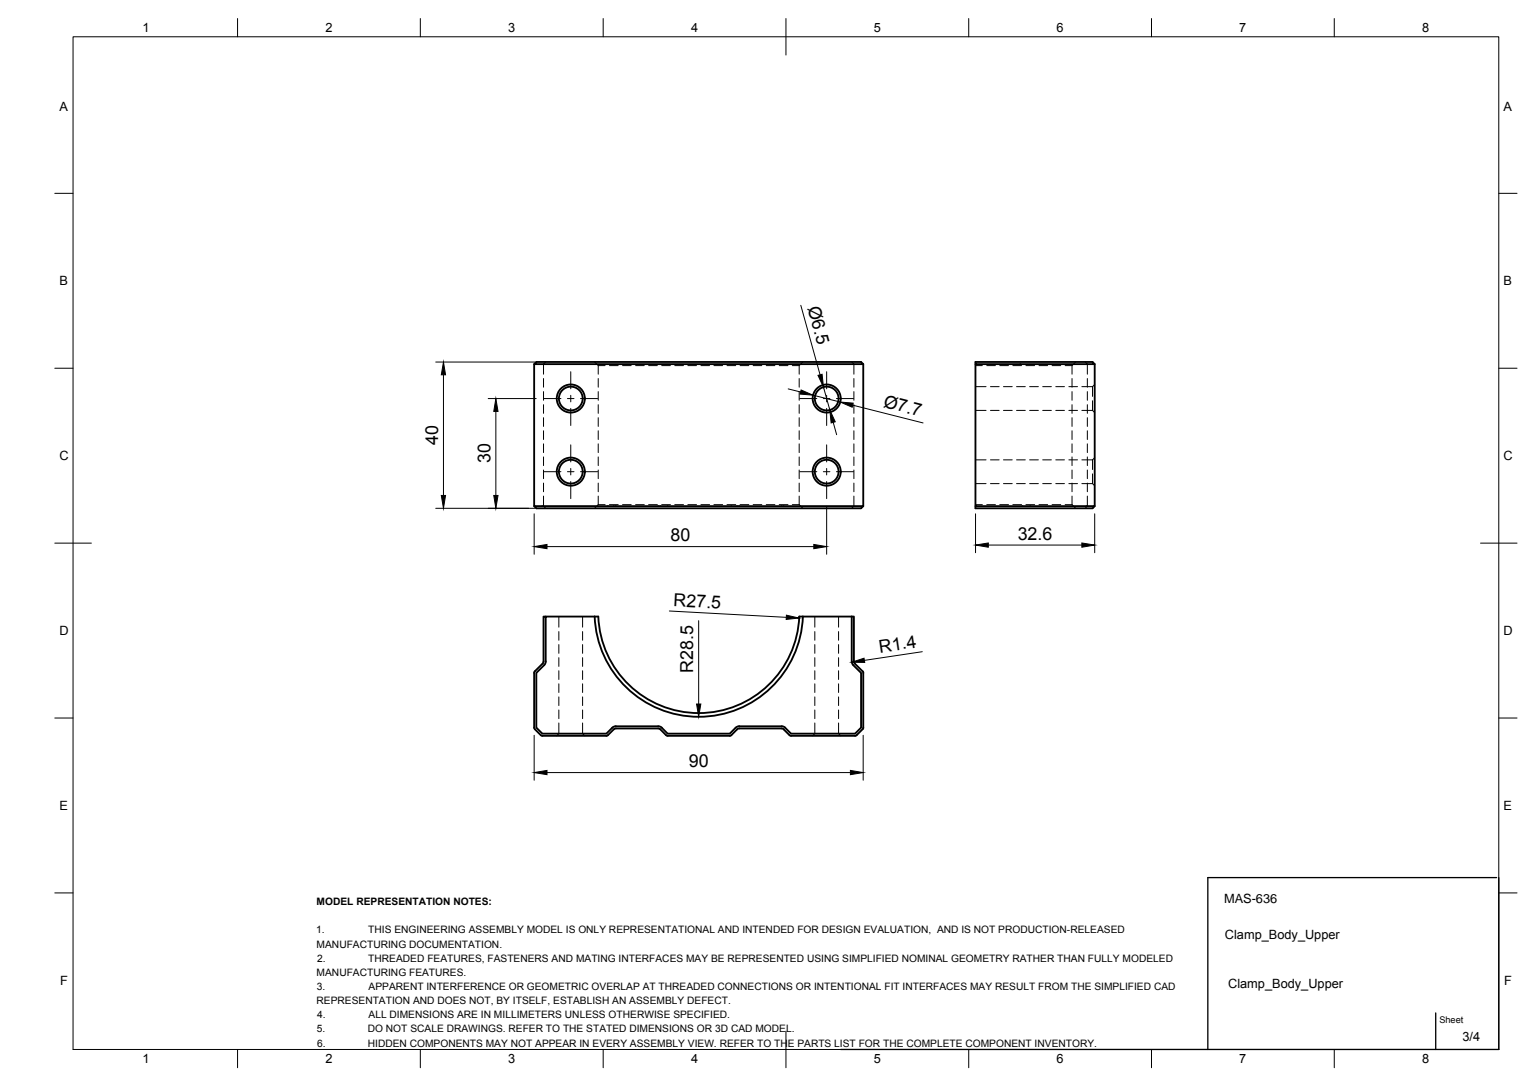
ISO-10303-21;
HEADER;
FILE_DESCRIPTION((''),'2;1');
FILE_NAME('Clamp_Body_Upper.step','2026-10-09T10:15:02-07:00',(''),(''),'','','');
FILE_SCHEMA (('AUTOMOTIVE_DESIGN { 1 0 10303 214 3 1 1 }'));
ENDSEC;
DATA;
#10=MECHANICAL_DESIGN_GEOMETRIC_PRESENTATION_REPRESENTATION('',(#83),#6779);
#63=SHAPE_REPRESENTATION_RELATIONSHIP('SRR','None',#6817,#73) ;
#73=ADVANCED_BREP_SHAPE_REPRESENTATION('',(#93),#6769) ;
#83=STYLED_ITEM('',(#6876),#93) ;
#93=MANIFOLD_SOLID_BREP('Body1',#3895) ;
#103=FACE_BOUND('',#628,.T.) ;
#104=FACE_BOUND('',#629,.T.) ;
#105=FACE_BOUND('',#631,.T.) ;
#106=FACE_BOUND('',#632,.T.) ;
#107=FACE_BOUND('',#638,.T.) ;
#108=FACE_BOUND('',#639,.T.) ;
#109=FACE_BOUND('',#649,.T.) ;
#110=FACE_BOUND('',#650,.T.) ;
#135=PLANE('',#4045) ;
#136=PLANE('',#4054) ;
#137=PLANE('',#4057) ;
#138=PLANE('',#4060) ;
#139=PLANE('',#4063) ;
#140=PLANE('',#4066) ;
#141=PLANE('',#4069) ;
#142=PLANE('',#4072) ;
#143=PLANE('',#4075) ;
#144=PLANE('',#4078) ;
#145=PLANE('',#4081) ;
#146=PLANE('',#4084) ;
#147=PLANE('',#4087) ;
#148=PLANE('',#4090) ;
#149=PLANE('',#4093) ;
#150=PLANE('',#4096) ;
#151=PLANE('',#4099) ;
#152=PLANE('',#4100) ;
#153=PLANE('',#4101) ;
#154=PLANE('',#4120) ;
#155=PLANE('',#4121) ;
#156=PLANE('',#4122) ;
#157=PLANE('',#4123) ;
#158=PLANE('',#4124) ;
#159=PLANE('',#4125) ;
#160=PLANE('',#4128) ;
#161=PLANE('',#4131) ;
#162=PLANE('',#4132) ;
#163=PLANE('',#4135) ;
#164=PLANE('',#4138) ;
#165=PLANE('',#4139) ;
#166=PLANE('',#4142) ;
#167=PLANE('',#4145) ;
#168=PLANE('',#4148) ;
#169=PLANE('',#4151) ;
#170=PLANE('',#4152) ;
#171=PLANE('',#4155) ;
#172=PLANE('',#4156) ;
#173=PLANE('',#4160) ;
#174=PLANE('',#4162) ;
#175=PLANE('',#4164) ;
#176=PLANE('',#4166) ;
#177=PLANE('',#4168) ;
#178=PLANE('',#4170) ;
#179=PLANE('',#4172) ;
#180=PLANE('',#4174) ;
#181=PLANE('',#4176) ;
#182=PLANE('',#4178) ;
#183=PLANE('',#4180) ;
#184=PLANE('',#4182) ;
#185=PLANE('',#4184) ;
#186=PLANE('',#4186) ;
#187=PLANE('',#4188) ;
#188=PLANE('',#4190) ;
#189=PLANE('',#4191) ;
#263=(
BOUNDED_CURVE()
B_SPLINE_CURVE(2,(#5652,#5653,#5654),.UNSPECIFIED.,.F.,.F.)
B_SPLINE_CURVE_WITH_KNOTS((3,3),(8.17571637705571,8.18145882895963),
 .UNSPECIFIED.)
CURVE()
GEOMETRIC_REPRESENTATION_ITEM()
RATIONAL_B_SPLINE_CURVE((1.06993006993377,1.0518696293833,1.03378378378363))
REPRESENTATION_ITEM('')
) ;
#264=(
BOUNDED_CURVE()
B_SPLINE_CURVE(2,(#5656,#5657,#5658),.UNSPECIFIED.,.F.,.F.)
B_SPLINE_CURVE_WITH_KNOTS((3,3),(-0.0111022969227764,-0.00535984501964869),
 .UNSPECIFIED.)
CURVE()
GEOMETRIC_REPRESENTATION_ITEM()
RATIONAL_B_SPLINE_CURVE((1.06993006993377,1.0518696293858,1.03378378378863))
REPRESENTATION_ITEM('')
) ;
#265=(
BOUNDED_CURVE()
B_SPLINE_CURVE(2,(#5664,#5665,#5666),.UNSPECIFIED.,.F.,.F.)
B_SPLINE_CURVE_WITH_KNOTS((3,3),(8.1757163770557,8.18145882895962),
 .UNSPECIFIED.)
CURVE()
GEOMETRIC_REPRESENTATION_ITEM()
RATIONAL_B_SPLINE_CURVE((1.06993006993376,1.05186962938329,1.03378378378362))
REPRESENTATION_ITEM('')
) ;
#266=(
BOUNDED_CURVE()
B_SPLINE_CURVE(2,(#5667,#5668,#5669),.UNSPECIFIED.,.F.,.F.)
B_SPLINE_CURVE_WITH_KNOTS((3,3),(-0.0111022969227769,-0.00535984501964911),
 .UNSPECIFIED.)
CURVE()
GEOMETRIC_REPRESENTATION_ITEM()
RATIONAL_B_SPLINE_CURVE((1.06993006993377,1.0518696293858,1.03378378378863))
REPRESENTATION_ITEM('')
) ;
#267=CONICAL_SURFACE('',#4021,1.,0.785398163397) ;
#268=CONICAL_SURFACE('',#4023,1.,0.785398163397) ;
#269=CONICAL_SURFACE('',#4028,1.,0.785398163398) ;
#270=CONICAL_SURFACE('',#4033,1.,0.785398163398) ;
#271=CONICAL_SURFACE('',#4038,1.,0.785398163398) ;
#272=CONICAL_SURFACE('',#4043,1.,0.785398163398) ;
#273=CONICAL_SURFACE('',#4052,1.,0.785398163392) ;
#274=CONICAL_SURFACE('',#4055,1.,0.785398163397) ;
#275=CONICAL_SURFACE('',#4058,1.,0.785398163397) ;
#276=CONICAL_SURFACE('',#4061,1.,0.785398163397) ;
#277=CONICAL_SURFACE('',#4064,1.,0.785398163397) ;
#278=CONICAL_SURFACE('',#4067,1.,0.785398163392) ;
#279=CONICAL_SURFACE('',#4070,1.,0.785398163392) ;
#280=CONICAL_SURFACE('',#4073,1.,0.785398163397) ;
#281=CONICAL_SURFACE('',#4076,1.,0.785398163397) ;
#282=CONICAL_SURFACE('',#4079,1.,0.785398163397) ;
#283=CONICAL_SURFACE('',#4082,1.,0.785398163397) ;
#284=CONICAL_SURFACE('',#4085,1.,0.785398163397) ;
#285=CONICAL_SURFACE('',#4088,1.,0.785398163397) ;
#286=CONICAL_SURFACE('',#4091,1.,0.785398163397) ;
#287=CONICAL_SURFACE('',#4094,1.,0.785398163397) ;
#288=CONICAL_SURFACE('',#4097,1.,0.785398163397) ;
#289=CONICAL_SURFACE('',#4159,1.,0.785398163392) ;
#290=CONICAL_SURFACE('',#4161,1.,0.785398163397) ;
#291=CONICAL_SURFACE('',#4163,1.,0.785398163397) ;
#292=CONICAL_SURFACE('',#4165,1.,0.785398163397) ;
#293=CONICAL_SURFACE('',#4167,1.,0.785398163397) ;
#294=CONICAL_SURFACE('',#4169,1.,0.785398163372) ;
#295=CONICAL_SURFACE('',#4171,1.,0.785398163372) ;
#296=CONICAL_SURFACE('',#4173,1.,0.785398163397) ;
#297=CONICAL_SURFACE('',#4175,1.,0.785398163397) ;
#298=CONICAL_SURFACE('',#4177,1.,0.785398163397) ;
#299=CONICAL_SURFACE('',#4179,1.,0.785398163397) ;
#300=CONICAL_SURFACE('',#4181,1.,0.785398163397) ;
#301=CONICAL_SURFACE('',#4183,1.,0.785398163397) ;
#302=CONICAL_SURFACE('',#4185,1.,0.785398163397) ;
#303=CONICAL_SURFACE('',#4187,1.,0.785398163397) ;
#304=CONICAL_SURFACE('',#4189,1.,0.785398163397) ;
#327=FACE_OUTER_BOUND('',#571,.T.) ;
#328=FACE_OUTER_BOUND('',#572,.T.) ;
#329=FACE_OUTER_BOUND('',#573,.T.) ;
#330=FACE_OUTER_BOUND('',#574,.T.) ;
#331=FACE_OUTER_BOUND('',#575,.T.) ;
#332=FACE_OUTER_BOUND('',#576,.T.) ;
#333=FACE_OUTER_BOUND('',#577,.T.) ;
#334=FACE_OUTER_BOUND('',#578,.T.) ;
#335=FACE_OUTER_BOUND('',#579,.T.) ;
#336=FACE_OUTER_BOUND('',#580,.T.) ;
#337=FACE_OUTER_BOUND('',#581,.T.) ;
#338=FACE_OUTER_BOUND('',#582,.T.) ;
#339=FACE_OUTER_BOUND('',#583,.T.) ;
#340=FACE_OUTER_BOUND('',#584,.T.) ;
#341=FACE_OUTER_BOUND('',#585,.T.) ;
#342=FACE_OUTER_BOUND('',#586,.T.) ;
#343=FACE_OUTER_BOUND('',#587,.T.) ;
#344=FACE_OUTER_BOUND('',#588,.T.) ;
#345=FACE_OUTER_BOUND('',#589,.T.) ;
#346=FACE_OUTER_BOUND('',#590,.T.) ;
#347=FACE_OUTER_BOUND('',#591,.T.) ;
#348=FACE_OUTER_BOUND('',#592,.T.) ;
#349=FACE_OUTER_BOUND('',#593,.T.) ;
#350=FACE_OUTER_BOUND('',#594,.T.) ;
#351=FACE_OUTER_BOUND('',#595,.T.) ;
#352=FACE_OUTER_BOUND('',#596,.T.) ;
#353=FACE_OUTER_BOUND('',#597,.T.) ;
#354=FACE_OUTER_BOUND('',#598,.T.) ;
#355=FACE_OUTER_BOUND('',#599,.T.) ;
#356=FACE_OUTER_BOUND('',#600,.T.) ;
#357=FACE_OUTER_BOUND('',#601,.T.) ;
#358=FACE_OUTER_BOUND('',#602,.T.) ;
#359=FACE_OUTER_BOUND('',#603,.T.) ;
#360=FACE_OUTER_BOUND('',#604,.T.) ;
#361=FACE_OUTER_BOUND('',#605,.T.) ;
#362=FACE_OUTER_BOUND('',#606,.T.) ;
#363=FACE_OUTER_BOUND('',#607,.T.) ;
#364=FACE_OUTER_BOUND('',#608,.T.) ;
#365=FACE_OUTER_BOUND('',#609,.T.) ;
#366=FACE_OUTER_BOUND('',#610,.T.) ;
#367=FACE_OUTER_BOUND('',#611,.T.) ;
#368=FACE_OUTER_BOUND('',#612,.T.) ;
#369=FACE_OUTER_BOUND('',#613,.T.) ;
#370=FACE_OUTER_BOUND('',#614,.T.) ;
#371=FACE_OUTER_BOUND('',#615,.T.) ;
#372=FACE_OUTER_BOUND('',#616,.T.) ;
#373=FACE_OUTER_BOUND('',#617,.T.) ;
#374=FACE_OUTER_BOUND('',#618,.T.) ;
#375=FACE_OUTER_BOUND('',#619,.T.) ;
#376=FACE_OUTER_BOUND('',#620,.T.) ;
#377=FACE_OUTER_BOUND('',#621,.T.) ;
#378=FACE_OUTER_BOUND('',#622,.T.) ;
#379=FACE_OUTER_BOUND('',#623,.T.) ;
#380=FACE_OUTER_BOUND('',#624,.T.) ;
#381=FACE_OUTER_BOUND('',#625,.T.) ;
#382=FACE_OUTER_BOUND('',#626,.T.) ;
#383=FACE_OUTER_BOUND('',#627,.T.) ;
#384=FACE_OUTER_BOUND('',#630,.T.) ;
#385=FACE_OUTER_BOUND('',#633,.T.) ;
#386=FACE_OUTER_BOUND('',#634,.T.) ;
#387=FACE_OUTER_BOUND('',#635,.T.) ;
#388=FACE_OUTER_BOUND('',#636,.T.) ;
#389=FACE_OUTER_BOUND('',#637,.T.) ;
#390=FACE_OUTER_BOUND('',#640,.T.) ;
#391=FACE_OUTER_BOUND('',#641,.T.) ;
#392=FACE_OUTER_BOUND('',#642,.T.) ;
#393=FACE_OUTER_BOUND('',#643,.T.) ;
#394=FACE_OUTER_BOUND('',#644,.T.) ;
#395=FACE_OUTER_BOUND('',#645,.T.) ;
#396=FACE_OUTER_BOUND('',#646,.T.) ;
#397=FACE_OUTER_BOUND('',#647,.T.) ;
#398=FACE_OUTER_BOUND('',#648,.T.) ;
#399=FACE_OUTER_BOUND('',#651,.T.) ;
#400=FACE_OUTER_BOUND('',#652,.T.) ;
#401=FACE_OUTER_BOUND('',#653,.T.) ;
#402=FACE_OUTER_BOUND('',#654,.T.) ;
#403=FACE_OUTER_BOUND('',#655,.T.) ;
#404=FACE_OUTER_BOUND('',#656,.T.) ;
#405=FACE_OUTER_BOUND('',#657,.T.) ;
#406=FACE_OUTER_BOUND('',#658,.T.) ;
#407=FACE_OUTER_BOUND('',#659,.T.) ;
#408=FACE_OUTER_BOUND('',#660,.T.) ;
#409=FACE_OUTER_BOUND('',#661,.T.) ;
#410=FACE_OUTER_BOUND('',#662,.T.) ;
#411=FACE_OUTER_BOUND('',#663,.T.) ;
#412=FACE_OUTER_BOUND('',#664,.T.) ;
#413=FACE_OUTER_BOUND('',#665,.T.) ;
#414=FACE_OUTER_BOUND('',#666,.T.) ;
#415=FACE_OUTER_BOUND('',#667,.T.) ;
#416=FACE_OUTER_BOUND('',#668,.T.) ;
#417=FACE_OUTER_BOUND('',#669,.T.) ;
#418=FACE_OUTER_BOUND('',#670,.T.) ;
#419=FACE_OUTER_BOUND('',#671,.T.) ;
#420=FACE_OUTER_BOUND('',#672,.T.) ;
#421=FACE_OUTER_BOUND('',#673,.T.) ;
#422=FACE_OUTER_BOUND('',#674,.T.) ;
#423=FACE_OUTER_BOUND('',#675,.T.) ;
#424=FACE_OUTER_BOUND('',#676,.T.) ;
#425=FACE_OUTER_BOUND('',#677,.T.) ;
#426=FACE_OUTER_BOUND('',#678,.T.) ;
#427=FACE_OUTER_BOUND('',#679,.T.) ;
#428=FACE_OUTER_BOUND('',#680,.T.) ;
#429=FACE_OUTER_BOUND('',#681,.T.) ;
#430=FACE_OUTER_BOUND('',#682,.T.) ;
#431=FACE_OUTER_BOUND('',#683,.T.) ;
#432=FACE_OUTER_BOUND('',#684,.T.) ;
#433=FACE_OUTER_BOUND('',#685,.T.) ;
#434=FACE_OUTER_BOUND('',#686,.T.) ;
#435=FACE_OUTER_BOUND('',#687,.T.) ;
#436=FACE_OUTER_BOUND('',#688,.T.) ;
#437=FACE_OUTER_BOUND('',#689,.T.) ;
#438=FACE_OUTER_BOUND('',#690,.T.) ;
#439=FACE_OUTER_BOUND('',#691,.T.) ;
#440=FACE_OUTER_BOUND('',#692,.T.) ;
#571=EDGE_LOOP('',(#2555,#2556,#2557,#2558)) ;
#572=EDGE_LOOP('',(#2559,#2560,#2561,#2562)) ;
#573=EDGE_LOOP('',(#2563,#2564,#2565,#2566)) ;
#574=EDGE_LOOP('',(#2567,#2568,#2569,#2570)) ;
#575=EDGE_LOOP('',(#2571,#2572,#2573,#2574)) ;
#576=EDGE_LOOP('',(#2575,#2576,#2577,#2578)) ;
#577=EDGE_LOOP('',(#2579,#2580,#2581,#2582)) ;
#578=EDGE_LOOP('',(#2583,#2584,#2585,#2586)) ;
#579=EDGE_LOOP('',(#2587,#2588,#2589,#2590)) ;
#580=EDGE_LOOP('',(#2591,#2592,#2593,#2594)) ;
#581=EDGE_LOOP('',(#2595,#2596,#2597,#2598)) ;
#582=EDGE_LOOP('',(#2599,#2600,#2601,#2602,#2603,#2604,#2605,#2606,#2607,
#2608,#2609,#2610,#2611,#2612,#2613,#2614,#2615,#2616,#2617,#2618,#2619,
#2620,#2621,#2622,#2623,#2624)) ;
#583=EDGE_LOOP('',(#2625,#2626,#2627,#2628)) ;
#584=EDGE_LOOP('',(#2629,#2630,#2631,#2632)) ;
#585=EDGE_LOOP('',(#2633,#2634,#2635)) ;
#586=EDGE_LOOP('',(#2636,#2637,#2638,#2639)) ;
#587=EDGE_LOOP('',(#2640,#2641,#2642)) ;
#588=EDGE_LOOP('',(#2643,#2644,#2645,#2646)) ;
#589=EDGE_LOOP('',(#2647,#2648,#2649)) ;
#590=EDGE_LOOP('',(#2650,#2651,#2652,#2653)) ;
#591=EDGE_LOOP('',(#2654,#2655,#2656)) ;
#592=EDGE_LOOP('',(#2657,#2658,#2659,#2660)) ;
#593=EDGE_LOOP('',(#2661,#2662,#2663,#2664)) ;
#594=EDGE_LOOP('',(#2665,#2666,#2667,#2668)) ;
#595=EDGE_LOOP('',(#2669,#2670,#2671,#2672)) ;
#596=EDGE_LOOP('',(#2673,#2674,#2675,#2676)) ;
#597=EDGE_LOOP('',(#2677,#2678,#2679)) ;
#598=EDGE_LOOP('',(#2680,#2681,#2682,#2683)) ;
#599=EDGE_LOOP('',(#2684,#2685,#2686)) ;
#600=EDGE_LOOP('',(#2687,#2688,#2689,#2690)) ;
#601=EDGE_LOOP('',(#2691,#2692,#2693,#2694)) ;
#602=EDGE_LOOP('',(#2695,#2696,#2697,#2698)) ;
#603=EDGE_LOOP('',(#2699,#2700,#2701,#2702)) ;
#604=EDGE_LOOP('',(#2703,#2704,#2705,#2706)) ;
#605=EDGE_LOOP('',(#2707,#2708,#2709)) ;
#606=EDGE_LOOP('',(#2710,#2711,#2712,#2713)) ;
#607=EDGE_LOOP('',(#2714,#2715,#2716)) ;
#608=EDGE_LOOP('',(#2717,#2718,#2719,#2720)) ;
#609=EDGE_LOOP('',(#2721,#2722,#2723)) ;
#610=EDGE_LOOP('',(#2724,#2725,#2726,#2727)) ;
#611=EDGE_LOOP('',(#2728,#2729,#2730)) ;
#612=EDGE_LOOP('',(#2731,#2732,#2733,#2734)) ;
#613=EDGE_LOOP('',(#2735,#2736,#2737,#2738)) ;
#614=EDGE_LOOP('',(#2739,#2740,#2741,#2742)) ;
#615=EDGE_LOOP('',(#2743,#2744,#2745,#2746)) ;
#616=EDGE_LOOP('',(#2747,#2748,#2749,#2750,#2751,#2752,#2753,#2754,#2755,
#2756,#2757,#2758,#2759,#2760,#2761,#2762,#2763,#2764,#2765,#2766,#2767,
#2768,#2769,#2770,#2771,#2772)) ;
#617=EDGE_LOOP('',(#2773,#2774,#2775,#2776)) ;
#618=EDGE_LOOP('',(#2777,#2778,#2779,#2780)) ;
#619=EDGE_LOOP('',(#2781,#2782,#2783,#2784)) ;
#620=EDGE_LOOP('',(#2785,#2786,#2787,#2788)) ;
#621=EDGE_LOOP('',(#2789,#2790,#2791,#2792)) ;
#622=EDGE_LOOP('',(#2793,#2794,#2795,#2796)) ;
#623=EDGE_LOOP('',(#2797,#2798,#2799,#2800)) ;
#624=EDGE_LOOP('',(#2801,#2802,#2803,#2804)) ;
#625=EDGE_LOOP('',(#2805,#2806,#2807,#2808)) ;
#626=EDGE_LOOP('',(#2809,#2810,#2811,#2812)) ;
#627=EDGE_LOOP('',(#2813,#2814,#2815,#2816,#2817,#2818,#2819,#2820)) ;
#628=EDGE_LOOP('',(#2821)) ;
#629=EDGE_LOOP('',(#2822)) ;
#630=EDGE_LOOP('',(#2823,#2824,#2825,#2826,#2827,#2828,#2829,#2830)) ;
#631=EDGE_LOOP('',(#2831)) ;
#632=EDGE_LOOP('',(#2832)) ;
#633=EDGE_LOOP('',(#2833,#2834,#2835,#2836)) ;
#634=EDGE_LOOP('',(#2837,#2838,#2839,#2840)) ;
#635=EDGE_LOOP('',(#2841,#2842,#2843,#2844)) ;
#636=EDGE_LOOP('',(#2845,#2846,#2847,#2848)) ;
#637=EDGE_LOOP('',(#2849,#2850,#2851,#2852)) ;
#638=EDGE_LOOP('',(#2853)) ;
#639=EDGE_LOOP('',(#2854)) ;
#640=EDGE_LOOP('',(#2855,#2856,#2857,#2858)) ;
#641=EDGE_LOOP('',(#2859,#2860,#2861,#2862)) ;
#642=EDGE_LOOP('',(#2863,#2864,#2865,#2866)) ;
#643=EDGE_LOOP('',(#2867,#2868,#2869,#2870)) ;
#644=EDGE_LOOP('',(#2871,#2872,#2873,#2874)) ;
#645=EDGE_LOOP('',(#2875,#2876,#2877,#2878)) ;
#646=EDGE_LOOP('',(#2879,#2880,#2881,#2882)) ;
#647=EDGE_LOOP('',(#2883,#2884,#2885,#2886)) ;
#648=EDGE_LOOP('',(#2887,#2888,#2889,#2890)) ;
#649=EDGE_LOOP('',(#2891)) ;
#650=EDGE_LOOP('',(#2892)) ;
#651=EDGE_LOOP('',(#2893,#2894,#2895,#2896)) ;
#652=EDGE_LOOP('',(#2897,#2898,#2899,#2900)) ;
#653=EDGE_LOOP('',(#2901,#2902,#2903,#2904)) ;
#654=EDGE_LOOP('',(#2905,#2906,#2907,#2908)) ;
#655=EDGE_LOOP('',(#2909,#2910,#2911,#2912)) ;
#656=EDGE_LOOP('',(#2913,#2914,#2915,#2916)) ;
#657=EDGE_LOOP('',(#2917,#2918,#2919,#2920)) ;
#658=EDGE_LOOP('',(#2921,#2922,#2923,#2924)) ;
#659=EDGE_LOOP('',(#2925,#2926,#2927,#2928)) ;
#660=EDGE_LOOP('',(#2929,#2930,#2931,#2932)) ;
#661=EDGE_LOOP('',(#2933,#2934,#2935,#2936)) ;
#662=EDGE_LOOP('',(#2937,#2938,#2939)) ;
#663=EDGE_LOOP('',(#2940,#2941,#2942,#2943)) ;
#664=EDGE_LOOP('',(#2944,#2945,#2946)) ;
#665=EDGE_LOOP('',(#2947,#2948,#2949,#2950)) ;
#666=EDGE_LOOP('',(#2951,#2952,#2953)) ;
#667=EDGE_LOOP('',(#2954,#2955,#2956,#2957)) ;
#668=EDGE_LOOP('',(#2958,#2959,#2960)) ;
#669=EDGE_LOOP('',(#2961,#2962,#2963,#2964)) ;
#670=EDGE_LOOP('',(#2965,#2966,#2967,#2968)) ;
#671=EDGE_LOOP('',(#2969,#2970,#2971,#2972)) ;
#672=EDGE_LOOP('',(#2973,#2974,#2975,#2976)) ;
#673=EDGE_LOOP('',(#2977,#2978,#2979,#2980)) ;
#674=EDGE_LOOP('',(#2981,#2982,#2983)) ;
#675=EDGE_LOOP('',(#2984,#2985,#2986,#2987)) ;
#676=EDGE_LOOP('',(#2988,#2989,#2990)) ;
#677=EDGE_LOOP('',(#2991,#2992,#2993,#2994)) ;
#678=EDGE_LOOP('',(#2995,#2996,#2997,#2998)) ;
#679=EDGE_LOOP('',(#2999,#3000,#3001,#3002)) ;
#680=EDGE_LOOP('',(#3003,#3004,#3005,#3006)) ;
#681=EDGE_LOOP('',(#3007,#3008,#3009,#3010)) ;
#682=EDGE_LOOP('',(#3011,#3012,#3013)) ;
#683=EDGE_LOOP('',(#3014,#3015,#3016,#3017)) ;
#684=EDGE_LOOP('',(#3018,#3019,#3020)) ;
#685=EDGE_LOOP('',(#3021,#3022,#3023,#3024)) ;
#686=EDGE_LOOP('',(#3025,#3026,#3027)) ;
#687=EDGE_LOOP('',(#3028,#3029,#3030,#3031)) ;
#688=EDGE_LOOP('',(#3032,#3033,#3034)) ;
#689=EDGE_LOOP('',(#3035,#3036,#3037,#3038)) ;
#690=EDGE_LOOP('',(#3039,#3040,#3041,#3042)) ;
#691=EDGE_LOOP('',(#3043,#3044,#3045,#3046)) ;
#692=EDGE_LOOP('',(#3047,#3048,#3049,#3050)) ;
#847=LINE('',#5646,#1207) ;
#848=LINE('',#5649,#1208) ;
#849=LINE('',#5674,#1209) ;
#850=LINE('',#5678,#1210) ;
#851=LINE('',#5684,#1211) ;
#852=LINE('',#5688,#1212) ;
#853=LINE('',#5694,#1213) ;
#854=LINE('',#5698,#1214) ;
#855=LINE('',#5704,#1215) ;
#856=LINE('',#5708,#1216) ;
#857=LINE('',#5712,#1217) ;
#858=LINE('',#5714,#1218) ;
#859=LINE('',#5716,#1219) ;
#860=LINE('',#5720,#1220) ;
#861=LINE('',#5722,#1221) ;
#862=LINE('',#5724,#1222) ;
#863=LINE('',#5726,#1223) ;
#864=LINE('',#5728,#1224) ;
#865=LINE('',#5732,#1225) ;
#866=LINE('',#5736,#1226) ;
#867=LINE('',#5738,#1227) ;
#868=LINE('',#5740,#1228) ;
#869=LINE('',#5744,#1229) ;
#870=LINE('',#5748,#1230) ;
#871=LINE('',#5750,#1231) ;
#872=LINE('',#5752,#1232) ;
#873=LINE('',#5754,#1233) ;
#874=LINE('',#5756,#1234) ;
#875=LINE('',#5759,#1235) ;
#876=LINE('',#5762,#1236) ;
#877=LINE('',#5765,#1237) ;
#878=LINE('',#5768,#1238) ;
#879=LINE('',#5769,#1239) ;
#880=LINE('',#5773,#1240) ;
#881=LINE('',#5776,#1241) ;
#882=LINE('',#5777,#1242) ;
#883=LINE('',#5781,#1243) ;
#884=LINE('',#5784,#1244) ;
#885=LINE('',#5785,#1245) ;
#886=LINE('',#5789,#1246) ;
#887=LINE('',#5792,#1247) ;
#888=LINE('',#5793,#1248) ;
#889=LINE('',#5797,#1249) ;
#890=LINE('',#5800,#1250) ;
#891=LINE('',#5801,#1251) ;
#892=LINE('',#5805,#1252) ;
#893=LINE('',#5808,#1253) ;
#894=LINE('',#5809,#1254) ;
#895=LINE('',#5813,#1255) ;
#896=LINE('',#5816,#1256) ;
#897=LINE('',#5817,#1257) ;
#898=LINE('',#5821,#1258) ;
#899=LINE('',#5824,#1259) ;
#900=LINE('',#5825,#1260) ;
#901=LINE('',#5829,#1261) ;
#902=LINE('',#5832,#1262) ;
#903=LINE('',#5833,#1263) ;
#904=LINE('',#5837,#1264) ;
#905=LINE('',#5840,#1265) ;
#906=LINE('',#5841,#1266) ;
#907=LINE('',#5845,#1267) ;
#908=LINE('',#5848,#1268) ;
#909=LINE('',#5849,#1269) ;
#910=LINE('',#5853,#1270) ;
#911=LINE('',#5856,#1271) ;
#912=LINE('',#5857,#1272) ;
#913=LINE('',#5861,#1273) ;
#914=LINE('',#5864,#1274) ;
#915=LINE('',#5865,#1275) ;
#916=LINE('',#5869,#1276) ;
#917=LINE('',#5872,#1277) ;
#918=LINE('',#5873,#1278) ;
#919=LINE('',#5877,#1279) ;
#920=LINE('',#5880,#1280) ;
#921=LINE('',#5881,#1281) ;
#922=LINE('',#5885,#1282) ;
#923=LINE('',#5888,#1283) ;
#924=LINE('',#5889,#1284) ;
#925=LINE('',#5892,#1285) ;
#926=LINE('',#5893,#1286) ;
#927=LINE('',#5897,#1287) ;
#928=LINE('',#5901,#1288) ;
#929=LINE('',#5903,#1289) ;
#930=LINE('',#5905,#1290) ;
#931=LINE('',#5907,#1291) ;
#932=LINE('',#5909,#1292) ;
#933=LINE('',#5913,#1293) ;
#934=LINE('',#5917,#1294) ;
#935=LINE('',#5919,#1295) ;
#936=LINE('',#5921,#1296) ;
#937=LINE('',#5925,#1297) ;
#938=LINE('',#5929,#1298) ;
#939=LINE('',#5931,#1299) ;
#940=LINE('',#5933,#1300) ;
#941=LINE('',#5935,#1301) ;
#942=LINE('',#5937,#1302) ;
#943=LINE('',#5941,#1303) ;
#944=LINE('',#5942,#1304) ;
#945=LINE('',#5943,#1305) ;
#946=LINE('',#5948,#1306) ;
#947=LINE('',#5949,#1307) ;
#948=LINE('',#5954,#1308) ;
#949=LINE('',#5955,#1309) ;
#950=LINE('',#5960,#1310) ;
#951=LINE('',#5961,#1311) ;
#952=LINE('',#5966,#1312) ;
#953=LINE('',#5967,#1313) ;
#954=LINE('',#5972,#1314) ;
#955=LINE('',#5973,#1315) ;
#956=LINE('',#5978,#1316) ;
#957=LINE('',#5979,#1317) ;
#958=LINE('',#5982,#1318) ;
#959=LINE('',#5983,#1319) ;
#960=LINE('',#5985,#1320) ;
#961=LINE('',#5987,#1321) ;
#962=LINE('',#5990,#1322) ;
#963=LINE('',#5991,#1323) ;
#964=LINE('',#5993,#1324) ;
#965=LINE('',#5995,#1325) ;
#966=LINE('',#5998,#1326) ;
#967=LINE('',#6000,#1327) ;
#968=LINE('',#6004,#1328) ;
#969=LINE('',#6005,#1329) ;
#970=LINE('',#6008,#1330) ;
#971=LINE('',#6012,#1331) ;
#972=LINE('',#6013,#1332) ;
#973=LINE('',#6016,#1333) ;
#974=LINE('',#6017,#1334) ;
#975=LINE('',#6022,#1335) ;
#976=LINE('',#6023,#1336) ;
#977=LINE('',#6026,#1337) ;
#978=LINE('',#6030,#1338) ;
#979=LINE('',#6031,#1339) ;
#980=LINE('',#6034,#1340) ;
#981=LINE('',#6035,#1341) ;
#982=LINE('',#6040,#1342) ;
#983=LINE('',#6041,#1343) ;
#984=LINE('',#6044,#1344) ;
#985=LINE('',#6048,#1345) ;
#986=LINE('',#6049,#1346) ;
#987=LINE('',#6052,#1347) ;
#988=LINE('',#6056,#1348) ;
#989=LINE('',#6057,#1349) ;
#990=LINE('',#6060,#1350) ;
#991=LINE('',#6064,#1351) ;
#992=LINE('',#6065,#1352) ;
#993=LINE('',#6068,#1353) ;
#994=LINE('',#6069,#1354) ;
#995=LINE('',#6074,#1355) ;
#996=LINE('',#6075,#1356) ;
#997=LINE('',#6078,#1357) ;
#998=LINE('',#6079,#1358) ;
#999=LINE('',#6083,#1359) ;
#1000=LINE('',#6084,#1360) ;
#1001=LINE('',#6086,#1361) ;
#1002=LINE('',#6088,#1362) ;
#1003=LINE('',#6090,#1363) ;
#1004=LINE('',#6092,#1364) ;
#1005=LINE('',#6094,#1365) ;
#1006=LINE('',#6096,#1366) ;
#1007=LINE('',#6098,#1367) ;
#1008=LINE('',#6100,#1368) ;
#1009=LINE('',#6102,#1369) ;
#1010=LINE('',#6104,#1370) ;
#1011=LINE('',#6106,#1371) ;
#1012=LINE('',#6108,#1372) ;
#1013=LINE('',#6110,#1373) ;
#1014=LINE('',#6112,#1374) ;
#1015=LINE('',#6114,#1375) ;
#1016=LINE('',#6116,#1376) ;
#1017=LINE('',#6118,#1377) ;
#1018=LINE('',#6120,#1378) ;
#1019=LINE('',#6122,#1379) ;
#1020=LINE('',#6124,#1380) ;
#1021=LINE('',#6126,#1381) ;
#1022=LINE('',#6128,#1382) ;
#1023=LINE('',#6130,#1383) ;
#1024=LINE('',#6132,#1384) ;
#1025=LINE('',#6134,#1385) ;
#1026=LINE('',#6136,#1386) ;
#1027=LINE('',#6138,#1387) ;
#1028=LINE('',#6140,#1388) ;
#1029=LINE('',#6142,#1389) ;
#1030=LINE('',#6144,#1390) ;
#1207=VECTOR('',#4445,1.) ;
#1208=VECTOR('',#4448,1.) ;
#1209=VECTOR('',#4461,3.25) ;
#1210=VECTOR('',#4466,1.) ;
#1211=VECTOR('',#4473,3.25) ;
#1212=VECTOR('',#4478,1.) ;
#1213=VECTOR('',#4485,3.25) ;
#1214=VECTOR('',#4490,1.) ;
#1215=VECTOR('',#4497,3.25) ;
#1216=VECTOR('',#4502,1.) ;
#1217=VECTOR('',#4507,1.) ;
#1218=VECTOR('',#4508,1.) ;
#1219=VECTOR('',#4509,1.) ;
#1220=VECTOR('',#4512,1.00000000000064) ;
#1221=VECTOR('',#4513,1.) ;
#1222=VECTOR('',#4514,1.00000000000064) ;
#1223=VECTOR('',#4515,1.) ;
#1224=VECTOR('',#4516,1.00000000000064) ;
#1225=VECTOR('',#4519,1.) ;
#1226=VECTOR('',#4522,1.00000000000064) ;
#1227=VECTOR('',#4523,1.) ;
#1228=VECTOR('',#4524,1.00000000000064) ;
#1229=VECTOR('',#4527,1.) ;
#1230=VECTOR('',#4530,1.00000000000064) ;
#1231=VECTOR('',#4531,1.) ;
#1232=VECTOR('',#4532,1.00000000000064) ;
#1233=VECTOR('',#4533,1.) ;
#1234=VECTOR('',#4534,1.00000000000064) ;
#1235=VECTOR('',#4537,1.) ;
#1236=VECTOR('',#4540,0.999999999999933) ;
#1237=VECTOR('',#4543,0.99999999999982) ;
#1238=VECTOR('',#4546,1.00000000000064) ;
#1239=VECTOR('',#4547,1.00000000000032) ;
#1240=VECTOR('',#4552,1.00000000000064) ;
#1241=VECTOR('',#4555,1.) ;
#1242=VECTOR('',#4556,1.00000000000064) ;
#1243=VECTOR('',#4561,1.00000000000032) ;
#1244=VECTOR('',#4564,1.00000000000064) ;
#1245=VECTOR('',#4565,1.00000000000032) ;
#1246=VECTOR('',#4570,1.00000000000064) ;
#1247=VECTOR('',#4573,1.) ;
#1248=VECTOR('',#4574,1.00000000000064) ;
#1249=VECTOR('',#4579,1.00000000000032) ;
#1250=VECTOR('',#4582,1.00000000000064) ;
#1251=VECTOR('',#4583,1.00000000000032) ;
#1252=VECTOR('',#4588,0.999999999999933) ;
#1253=VECTOR('',#4591,1.) ;
#1254=VECTOR('',#4592,1.00000000000064) ;
#1255=VECTOR('',#4597,0.99999999999982) ;
#1256=VECTOR('',#4600,1.00000000000064) ;
#1257=VECTOR('',#4601,1.00000000000032) ;
#1258=VECTOR('',#4606,1.00000000000064) ;
#1259=VECTOR('',#4609,1.) ;
#1260=VECTOR('',#4610,1.00000000000064) ;
#1261=VECTOR('',#4615,1.00000000000032) ;
#1262=VECTOR('',#4618,1.00000000000064) ;
#1263=VECTOR('',#4619,1.00000000000032) ;
#1264=VECTOR('',#4624,1.00000000000064) ;
#1265=VECTOR('',#4627,1.) ;
#1266=VECTOR('',#4628,1.00000000000064) ;
#1267=VECTOR('',#4633,1.00000000000032) ;
#1268=VECTOR('',#4636,1.00000000000064) ;
#1269=VECTOR('',#4637,1.00000000000032) ;
#1270=VECTOR('',#4642,1.00000000000064) ;
#1271=VECTOR('',#4645,1.) ;
#1272=VECTOR('',#4646,1.00000000000064) ;
#1273=VECTOR('',#4651,1.00000000000032) ;
#1274=VECTOR('',#4654,1.00000000000064) ;
#1275=VECTOR('',#4655,1.00000000000032) ;
#1276=VECTOR('',#4660,1.00000000000064) ;
#1277=VECTOR('',#4663,1.) ;
#1278=VECTOR('',#4664,1.00000000000064) ;
#1279=VECTOR('',#4669,1.00000000000032) ;
#1280=VECTOR('',#4672,1.00000000000064) ;
#1281=VECTOR('',#4673,1.00000000000032) ;
#1282=VECTOR('',#4678,1.00000000000064) ;
#1283=VECTOR('',#4681,1.00000000000064) ;
#1284=VECTOR('',#4682,1.) ;
#1285=VECTOR('',#4685,1.) ;
#1286=VECTOR('',#4686,1.00000000000064) ;
#1287=VECTOR('',#4689,1.) ;
#1288=VECTOR('',#4692,1.00000000000064) ;
#1289=VECTOR('',#4693,1.) ;
#1290=VECTOR('',#4694,1.00000000000064) ;
#1291=VECTOR('',#4695,1.) ;
#1292=VECTOR('',#4696,1.00000000000064) ;
#1293=VECTOR('',#4699,1.) ;
#1294=VECTOR('',#4702,1.00000000000064) ;
#1295=VECTOR('',#4703,1.) ;
#1296=VECTOR('',#4704,1.00000000000064) ;
#1297=VECTOR('',#4707,1.) ;
#1298=VECTOR('',#4710,1.00000000000064) ;
#1299=VECTOR('',#4711,1.) ;
#1300=VECTOR('',#4712,1.00000000000064) ;
#1301=VECTOR('',#4713,1.) ;
#1302=VECTOR('',#4714,1.00000000000064) ;
#1303=VECTOR('',#4717,1.) ;
#1304=VECTOR('',#4718,1.) ;
#1305=VECTOR('',#4719,1.) ;
#1306=VECTOR('',#4724,1.) ;
#1307=VECTOR('',#4725,1.) ;
#1308=VECTOR('',#4730,1.) ;
#1309=VECTOR('',#4731,1.) ;
#1310=VECTOR('',#4736,1.) ;
#1311=VECTOR('',#4737,1.) ;
#1312=VECTOR('',#4742,1.) ;
#1313=VECTOR('',#4743,1.) ;
#1314=VECTOR('',#4748,1.) ;
#1315=VECTOR('',#4749,1.) ;
#1316=VECTOR('',#4754,1.) ;
#1317=VECTOR('',#4755,1.) ;
#1318=VECTOR('',#4758,1.) ;
#1319=VECTOR('',#4759,1.) ;
#1320=VECTOR('',#4762,1.) ;
#1321=VECTOR('',#4765,1.) ;
#1322=VECTOR('',#4768,1.) ;
#1323=VECTOR('',#4769,1.) ;
#1324=VECTOR('',#4772,1.00000000000064) ;
#1325=VECTOR('',#4775,1.00000000000064) ;
#1326=VECTOR('',#4778,1.) ;
#1327=VECTOR('',#4779,1.) ;
#1328=VECTOR('',#4784,1.) ;
#1329=VECTOR('',#4785,1.00000000000064) ;
#1330=VECTOR('',#4788,1.) ;
#1331=VECTOR('',#4793,1.) ;
#1332=VECTOR('',#4794,1.00000000000064) ;
#1333=VECTOR('',#4797,1.) ;
#1334=VECTOR('',#4798,1.) ;
#1335=VECTOR('',#4805,1.) ;
#1336=VECTOR('',#4806,1.00000000000064) ;
#1337=VECTOR('',#4809,1.) ;
#1338=VECTOR('',#4814,1.00000000000064) ;
#1339=VECTOR('',#4815,1.) ;
#1340=VECTOR('',#4818,1.) ;
#1341=VECTOR('',#4819,1.) ;
#1342=VECTOR('',#4826,1.00000000000064) ;
#1343=VECTOR('',#4827,1.) ;
#1344=VECTOR('',#4830,1.) ;
#1345=VECTOR('',#4835,1.) ;
#1346=VECTOR('',#4836,1.) ;
#1347=VECTOR('',#4839,1.) ;
#1348=VECTOR('',#4844,1.00000000000064) ;
#1349=VECTOR('',#4845,1.) ;
#1350=VECTOR('',#4848,1.) ;
#1351=VECTOR('',#4853,1.00000000000064) ;
#1352=VECTOR('',#4854,1.) ;
#1353=VECTOR('',#4857,1.) ;
#1354=VECTOR('',#4858,1.) ;
#1355=VECTOR('',#4865,1.) ;
#1356=VECTOR('',#4866,1.00000000000064) ;
#1357=VECTOR('',#4869,1.) ;
#1358=VECTOR('',#4870,1.) ;
#1359=VECTOR('',#4877,0.999999999999938) ;
#1360=VECTOR('',#4878,1.00000000000032) ;
#1361=VECTOR('',#4881,1.00000000000032) ;
#1362=VECTOR('',#4884,1.00000000000064) ;
#1363=VECTOR('',#4887,1.00000000000064) ;
#1364=VECTOR('',#4890,1.00000000000032) ;
#1365=VECTOR('',#4893,1.00000000000032) ;
#1366=VECTOR('',#4896,1.00000000000064) ;
#1367=VECTOR('',#4899,1.00000000000064) ;
#1368=VECTOR('',#4902,1.00000000000032) ;
#1369=VECTOR('',#4905,1.00000000000032) ;
#1370=VECTOR('',#4908,0.999999999999935) ;
#1371=VECTOR('',#4911,1.00000000000064) ;
#1372=VECTOR('',#4914,0.999999999999855) ;
#1373=VECTOR('',#4917,1.00000000000032) ;
#1374=VECTOR('',#4920,1.00000000000064) ;
#1375=VECTOR('',#4923,1.00000000000064) ;
#1376=VECTOR('',#4926,1.00000000000032) ;
#1377=VECTOR('',#4929,1.00000000000032) ;
#1378=VECTOR('',#4932,1.00000000000064) ;
#1379=VECTOR('',#4935,1.00000000000064) ;
#1380=VECTOR('',#4938,1.00000000000032) ;
#1381=VECTOR('',#4941,1.00000000000032) ;
#1382=VECTOR('',#4944,1.00000000000064) ;
#1383=VECTOR('',#4947,1.00000000000064) ;
#1384=VECTOR('',#4950,1.00000000000032) ;
#1385=VECTOR('',#4953,1.00000000000032) ;
#1386=VECTOR('',#4956,1.00000000000064) ;
#1387=VECTOR('',#4959,1.00000000000064) ;
#1388=VECTOR('',#4962,1.00000000000032) ;
#1389=VECTOR('',#4965,1.00000000000032) ;
#1390=VECTOR('',#4968,1.00000000000064) ;
#1567=CIRCLE('',#4019,27.5) ;
#1568=CIRCLE('',#4020,27.5) ;
#1569=CIRCLE('',#4022,28.5) ;
#1570=CIRCLE('',#4024,28.5) ;
#1571=CIRCLE('',#4026,3.25) ;
#1572=CIRCLE('',#4027,3.25) ;
#1573=CIRCLE('',#4029,3.85) ;
#1574=CIRCLE('',#4031,3.25) ;
#1575=CIRCLE('',#4032,3.25) ;
#1576=CIRCLE('',#4034,3.85) ;
#1577=CIRCLE('',#4036,3.25) ;
#1578=CIRCLE('',#4037,3.25) ;
#1579=CIRCLE('',#4039,3.85) ;
#1580=CIRCLE('',#4041,3.25) ;
#1581=CIRCLE('',#4042,3.25) ;
#1582=CIRCLE('',#4044,3.85) ;
#1583=CIRCLE('',#4046,1.39999840949753) ;
#1584=CIRCLE('',#4047,1.39999840966918) ;
#1585=CIRCLE('',#4048,1.39999840952888) ;
#1586=CIRCLE('',#4049,1.39999901980282) ;
#1587=CIRCLE('',#4050,1.39999901983735) ;
#1588=CIRCLE('',#4051,1.39999901980293) ;
#1589=CIRCLE('',#4053,0.8) ;
#1590=CIRCLE('',#4056,0.6) ;
#1591=CIRCLE('',#4059,0.6) ;
#1592=CIRCLE('',#4062,0.6) ;
#1593=CIRCLE('',#4065,0.6) ;
#1594=CIRCLE('',#4068,0.8) ;
#1595=CIRCLE('',#4071,0.8) ;
#1596=CIRCLE('',#4074,0.6) ;
#1597=CIRCLE('',#4077,0.6) ;
#1598=CIRCLE('',#4080,0.8) ;
#1599=CIRCLE('',#4083,0.8) ;
#1600=CIRCLE('',#4086,0.6) ;
#1601=CIRCLE('',#4089,0.6) ;
#1602=CIRCLE('',#4092,0.6) ;
#1603=CIRCLE('',#4095,0.6) ;
#1604=CIRCLE('',#4098,0.8) ;
#1605=CIRCLE('',#4102,1.39999901980304) ;
#1606=CIRCLE('',#4103,1.39999901983726) ;
#1607=CIRCLE('',#4104,1.39999901980286) ;
#1608=CIRCLE('',#4105,1.39999840950088) ;
#1609=CIRCLE('',#4106,1.39999840964119) ;
#1610=CIRCLE('',#4107,1.39999840949753) ;
#1611=CIRCLE('',#4109,0.8) ;
#1612=CIRCLE('',#4111,0.8) ;
#1613=CIRCLE('',#4113,0.8) ;
#1614=CIRCLE('',#4115,0.8) ;
#1615=CIRCLE('',#4117,0.8) ;
#1616=CIRCLE('',#4119,0.8) ;
#1617=CIRCLE('',#4127,0.6) ;
#1618=CIRCLE('',#4130,0.6) ;
#1619=CIRCLE('',#4134,0.6) ;
#1620=CIRCLE('',#4137,0.6) ;
#1621=CIRCLE('',#4141,0.6) ;
#1622=CIRCLE('',#4144,0.6) ;
#1623=CIRCLE('',#4147,0.6) ;
#1624=CIRCLE('',#4150,0.6) ;
#1625=CIRCLE('',#4154,0.6) ;
#1626=CIRCLE('',#4158,0.6) ;
#1723=VERTEX_POINT('',#5642) ;
#1724=VERTEX_POINT('',#5643) ;
#1725=VERTEX_POINT('',#5645) ;
#1726=VERTEX_POINT('',#5647) ;
#1727=VERTEX_POINT('',#5651) ;
#1728=VERTEX_POINT('',#5655) ;
#1729=VERTEX_POINT('',#5661) ;
#1730=VERTEX_POINT('',#5662) ;
#1731=VERTEX_POINT('',#5671) ;
#1732=VERTEX_POINT('',#5673) ;
#1733=VERTEX_POINT('',#5677) ;
#1734=VERTEX_POINT('',#5681) ;
#1735=VERTEX_POINT('',#5683) ;
#1736=VERTEX_POINT('',#5687) ;
#1737=VERTEX_POINT('',#5691) ;
#1738=VERTEX_POINT('',#5693) ;
#1739=VERTEX_POINT('',#5697) ;
#1740=VERTEX_POINT('',#5701) ;
#1741=VERTEX_POINT('',#5703) ;
#1742=VERTEX_POINT('',#5707) ;
#1743=VERTEX_POINT('',#5711) ;
#1744=VERTEX_POINT('',#5713) ;
#1745=VERTEX_POINT('',#5715) ;
#1746=VERTEX_POINT('',#5717) ;
#1747=VERTEX_POINT('',#5719) ;
#1748=VERTEX_POINT('',#5721) ;
#1749=VERTEX_POINT('',#5723) ;
#1750=VERTEX_POINT('',#5725) ;
#1751=VERTEX_POINT('',#5727) ;
#1752=VERTEX_POINT('',#5729) ;
#1753=VERTEX_POINT('',#5731) ;
#1754=VERTEX_POINT('',#5733) ;
#1755=VERTEX_POINT('',#5735) ;
#1756=VERTEX_POINT('',#5737) ;
#1757=VERTEX_POINT('',#5739) ;
#1758=VERTEX_POINT('',#5741) ;
#1759=VERTEX_POINT('',#5743) ;
#1760=VERTEX_POINT('',#5745) ;
#1761=VERTEX_POINT('',#5747) ;
#1762=VERTEX_POINT('',#5749) ;
#1763=VERTEX_POINT('',#5751) ;
#1764=VERTEX_POINT('',#5753) ;
#1765=VERTEX_POINT('',#5755) ;
#1766=VERTEX_POINT('',#5757) ;
#1767=VERTEX_POINT('',#5761) ;
#1768=VERTEX_POINT('',#5763) ;
#1769=VERTEX_POINT('',#5767) ;
#1770=VERTEX_POINT('',#5771) ;
#1771=VERTEX_POINT('',#5775) ;
#1772=VERTEX_POINT('',#5779) ;
#1773=VERTEX_POINT('',#5783) ;
#1774=VERTEX_POINT('',#5787) ;
#1775=VERTEX_POINT('',#5791) ;
#1776=VERTEX_POINT('',#5795) ;
#1777=VERTEX_POINT('',#5799) ;
#1778=VERTEX_POINT('',#5803) ;
#1779=VERTEX_POINT('',#5807) ;
#1780=VERTEX_POINT('',#5811) ;
#1781=VERTEX_POINT('',#5815) ;
#1782=VERTEX_POINT('',#5819) ;
#1783=VERTEX_POINT('',#5823) ;
#1784=VERTEX_POINT('',#5827) ;
#1785=VERTEX_POINT('',#5831) ;
#1786=VERTEX_POINT('',#5835) ;
#1787=VERTEX_POINT('',#5839) ;
#1788=VERTEX_POINT('',#5843) ;
#1789=VERTEX_POINT('',#5847) ;
#1790=VERTEX_POINT('',#5851) ;
#1791=VERTEX_POINT('',#5855) ;
#1792=VERTEX_POINT('',#5859) ;
#1793=VERTEX_POINT('',#5863) ;
#1794=VERTEX_POINT('',#5867) ;
#1795=VERTEX_POINT('',#5871) ;
#1796=VERTEX_POINT('',#5875) ;
#1797=VERTEX_POINT('',#5879) ;
#1798=VERTEX_POINT('',#5883) ;
#1799=VERTEX_POINT('',#5887) ;
#1800=VERTEX_POINT('',#5891) ;
#1801=VERTEX_POINT('',#5895) ;
#1802=VERTEX_POINT('',#5896) ;
#1803=VERTEX_POINT('',#5898) ;
#1804=VERTEX_POINT('',#5900) ;
#1805=VERTEX_POINT('',#5902) ;
#1806=VERTEX_POINT('',#5904) ;
#1807=VERTEX_POINT('',#5906) ;
#1808=VERTEX_POINT('',#5908) ;
#1809=VERTEX_POINT('',#5910) ;
#1810=VERTEX_POINT('',#5912) ;
#1811=VERTEX_POINT('',#5914) ;
#1812=VERTEX_POINT('',#5916) ;
#1813=VERTEX_POINT('',#5918) ;
#1814=VERTEX_POINT('',#5920) ;
#1815=VERTEX_POINT('',#5922) ;
#1816=VERTEX_POINT('',#5924) ;
#1817=VERTEX_POINT('',#5926) ;
#1818=VERTEX_POINT('',#5928) ;
#1819=VERTEX_POINT('',#5930) ;
#1820=VERTEX_POINT('',#5932) ;
#1821=VERTEX_POINT('',#5934) ;
#1822=VERTEX_POINT('',#5936) ;
#1823=VERTEX_POINT('',#5938) ;
#1824=VERTEX_POINT('',#5940) ;
#1825=VERTEX_POINT('',#5945) ;
#1826=VERTEX_POINT('',#5946) ;
#1827=VERTEX_POINT('',#5951) ;
#1828=VERTEX_POINT('',#5952) ;
#1829=VERTEX_POINT('',#5957) ;
#1830=VERTEX_POINT('',#5958) ;
#1831=VERTEX_POINT('',#5963) ;
#1832=VERTEX_POINT('',#5964) ;
#1833=VERTEX_POINT('',#5969) ;
#1834=VERTEX_POINT('',#5970) ;
#1835=VERTEX_POINT('',#5975) ;
#1836=VERTEX_POINT('',#5976) ;
#1837=VERTEX_POINT('',#5981) ;
#1838=VERTEX_POINT('',#5989) ;
#1839=VERTEX_POINT('',#5997) ;
#1840=VERTEX_POINT('',#5999) ;
#1841=VERTEX_POINT('',#6003) ;
#1842=VERTEX_POINT('',#6007) ;
#1843=VERTEX_POINT('',#6011) ;
#1844=VERTEX_POINT('',#6015) ;
#1845=VERTEX_POINT('',#6021) ;
#1846=VERTEX_POINT('',#6025) ;
#1847=VERTEX_POINT('',#6029) ;
#1848=VERTEX_POINT('',#6033) ;
#1849=VERTEX_POINT('',#6039) ;
#1850=VERTEX_POINT('',#6043) ;
#1851=VERTEX_POINT('',#6047) ;
#1852=VERTEX_POINT('',#6051) ;
#1853=VERTEX_POINT('',#6055) ;
#1854=VERTEX_POINT('',#6059) ;
#1855=VERTEX_POINT('',#6063) ;
#1856=VERTEX_POINT('',#6067) ;
#1857=VERTEX_POINT('',#6073) ;
#1858=VERTEX_POINT('',#6077) ;
#2031=EDGE_CURVE('',#1723,#1724,#1567,.F.) ;
#2032=EDGE_CURVE('',#1724,#1725,#847,.T.) ;
#2033=EDGE_CURVE('',#1726,#1725,#1568,.F.) ;
#2034=EDGE_CURVE('',#1723,#1726,#848,.T.) ;
#2035=EDGE_CURVE('',#1727,#1724,#263,.F.) ;
#2036=EDGE_CURVE('',#1723,#1728,#264,.T.) ;
#2037=EDGE_CURVE('',#1728,#1727,#1569,.F.) ;
#2038=EDGE_CURVE('',#1729,#1730,#1570,.F.) ;
#2039=EDGE_CURVE('',#1729,#1726,#265,.F.) ;
#2040=EDGE_CURVE('',#1725,#1730,#266,.T.) ;
#2041=EDGE_CURVE('',#1731,#1731,#1571,.F.) ;
#2042=EDGE_CURVE('',#1731,#1732,#849,.T.) ;
#2043=EDGE_CURVE('',#1732,#1732,#1572,.T.) ;
#2044=EDGE_CURVE('',#1732,#1733,#850,.T.) ;
#2045=EDGE_CURVE('',#1733,#1733,#1573,.T.) ;
#2046=EDGE_CURVE('',#1734,#1734,#1574,.F.) ;
#2047=EDGE_CURVE('',#1734,#1735,#851,.T.) ;
#2048=EDGE_CURVE('',#1735,#1735,#1575,.T.) ;
#2049=EDGE_CURVE('',#1735,#1736,#852,.T.) ;
#2050=EDGE_CURVE('',#1736,#1736,#1576,.T.) ;
#2051=EDGE_CURVE('',#1737,#1737,#1577,.F.) ;
#2052=EDGE_CURVE('',#1737,#1738,#853,.T.) ;
#2053=EDGE_CURVE('',#1738,#1738,#1578,.T.) ;
#2054=EDGE_CURVE('',#1738,#1739,#854,.T.) ;
#2055=EDGE_CURVE('',#1739,#1739,#1579,.T.) ;
#2056=EDGE_CURVE('',#1740,#1740,#1580,.F.) ;
#2057=EDGE_CURVE('',#1740,#1741,#855,.T.) ;
#2058=EDGE_CURVE('',#1741,#1741,#1581,.T.) ;
#2059=EDGE_CURVE('',#1741,#1742,#856,.T.) ;
#2060=EDGE_CURVE('',#1742,#1742,#1582,.T.) ;
#2061=EDGE_CURVE('',#1743,#1729,#857,.T.) ;
#2062=EDGE_CURVE('',#1730,#1744,#858,.F.) ;
#2063=EDGE_CURVE('',#1744,#1745,#859,.T.) ;
#2064=EDGE_CURVE('',#1745,#1746,#1583,.T.) ;
#2065=EDGE_CURVE('',#1746,#1747,#860,.T.) ;
#2066=EDGE_CURVE('',#1747,#1748,#861,.T.) ;
#2067=EDGE_CURVE('',#1748,#1749,#862,.F.) ;
#2068=EDGE_CURVE('',#1749,#1750,#863,.F.) ;
#2069=EDGE_CURVE('',#1750,#1751,#864,.F.) ;
#2070=EDGE_CURVE('',#1751,#1752,#1584,.T.) ;
#2071=EDGE_CURVE('',#1752,#1753,#865,.F.) ;
#2072=EDGE_CURVE('',#1753,#1754,#1585,.T.) ;
#2073=EDGE_CURVE('',#1754,#1755,#866,.F.) ;
#2074=EDGE_CURVE('',#1755,#1756,#867,.F.) ;
#2075=EDGE_CURVE('',#1756,#1757,#868,.T.) ;
#2076=EDGE_CURVE('',#1757,#1758,#1586,.T.) ;
#2077=EDGE_CURVE('',#1758,#1759,#869,.F.) ;
#2078=EDGE_CURVE('',#1759,#1760,#1587,.T.) ;
#2079=EDGE_CURVE('',#1760,#1761,#870,.T.) ;
#2080=EDGE_CURVE('',#1761,#1762,#871,.F.) ;
#2081=EDGE_CURVE('',#1762,#1763,#872,.T.) ;
#2082=EDGE_CURVE('',#1763,#1764,#873,.F.) ;
#2083=EDGE_CURVE('',#1764,#1765,#874,.F.) ;
#2084=EDGE_CURVE('',#1765,#1766,#1588,.T.) ;
#2085=EDGE_CURVE('',#1766,#1743,#875,.F.) ;
#2086=EDGE_CURVE('',#1745,#1767,#876,.F.) ;
#2087=EDGE_CURVE('',#1767,#1768,#1589,.T.) ;
#2088=EDGE_CURVE('',#1746,#1768,#877,.F.) ;
#2089=EDGE_CURVE('',#1768,#1769,#878,.T.) ;
#2090=EDGE_CURVE('',#1747,#1769,#879,.F.) ;
#2091=EDGE_CURVE('',#1769,#1770,#1590,.F.) ;
#2092=EDGE_CURVE('',#1747,#1770,#880,.T.) ;
#2093=EDGE_CURVE('',#1770,#1771,#881,.T.) ;
#2094=EDGE_CURVE('',#1748,#1771,#882,.F.) ;
#2095=EDGE_CURVE('',#1771,#1772,#1591,.F.) ;
#2096=EDGE_CURVE('',#1748,#1772,#883,.T.) ;
#2097=EDGE_CURVE('',#1772,#1773,#884,.F.) ;
#2098=EDGE_CURVE('',#1749,#1773,#885,.F.) ;
#2099=EDGE_CURVE('',#1773,#1774,#1592,.F.) ;
#2100=EDGE_CURVE('',#1749,#1774,#886,.T.) ;
#2101=EDGE_CURVE('',#1774,#1775,#887,.F.) ;
#2102=EDGE_CURVE('',#1750,#1775,#888,.F.) ;
#2103=EDGE_CURVE('',#1775,#1776,#1593,.F.) ;
#2104=EDGE_CURVE('',#1750,#1776,#889,.T.) ;
#2105=EDGE_CURVE('',#1776,#1777,#890,.F.) ;
#2106=EDGE_CURVE('',#1751,#1777,#891,.F.) ;
#2107=EDGE_CURVE('',#1777,#1778,#1594,.T.) ;
#2108=EDGE_CURVE('',#1752,#1778,#892,.F.) ;
#2109=EDGE_CURVE('',#1778,#1779,#893,.F.) ;
#2110=EDGE_CURVE('',#1753,#1779,#894,.F.) ;
#2111=EDGE_CURVE('',#1779,#1780,#1595,.T.) ;
#2112=EDGE_CURVE('',#1754,#1780,#895,.F.) ;
#2113=EDGE_CURVE('',#1780,#1781,#896,.F.) ;
#2114=EDGE_CURVE('',#1755,#1781,#897,.F.) ;
#2115=EDGE_CURVE('',#1781,#1782,#1596,.F.) ;
#2116=EDGE_CURVE('',#1755,#1782,#898,.T.) ;
#2117=EDGE_CURVE('',#1782,#1783,#899,.F.) ;
#2118=EDGE_CURVE('',#1756,#1783,#900,.F.) ;
#2119=EDGE_CURVE('',#1783,#1784,#1597,.F.) ;
#2120=EDGE_CURVE('',#1756,#1784,#901,.T.) ;
#2121=EDGE_CURVE('',#1784,#1785,#902,.T.) ;
#2122=EDGE_CURVE('',#1757,#1785,#903,.F.) ;
#2123=EDGE_CURVE('',#1785,#1786,#1598,.T.) ;
#2124=EDGE_CURVE('',#1758,#1786,#904,.F.) ;
#2125=EDGE_CURVE('',#1786,#1787,#905,.F.) ;
#2126=EDGE_CURVE('',#1759,#1787,#906,.F.) ;
#2127=EDGE_CURVE('',#1787,#1788,#1599,.T.) ;
#2128=EDGE_CURVE('',#1760,#1788,#907,.F.) ;
#2129=EDGE_CURVE('',#1788,#1789,#908,.T.) ;
#2130=EDGE_CURVE('',#1761,#1789,#909,.F.) ;
#2131=EDGE_CURVE('',#1789,#1790,#1600,.F.) ;
#2132=EDGE_CURVE('',#1761,#1790,#910,.T.) ;
#2133=EDGE_CURVE('',#1790,#1791,#911,.F.) ;
#2134=EDGE_CURVE('',#1762,#1791,#912,.F.) ;
#2135=EDGE_CURVE('',#1791,#1792,#1601,.F.) ;
#2136=EDGE_CURVE('',#1762,#1792,#913,.T.) ;
#2137=EDGE_CURVE('',#1792,#1793,#914,.T.) ;
#2138=EDGE_CURVE('',#1763,#1793,#915,.F.) ;
#2139=EDGE_CURVE('',#1793,#1794,#1602,.F.) ;
#2140=EDGE_CURVE('',#1763,#1794,#916,.T.) ;
#2141=EDGE_CURVE('',#1794,#1795,#917,.F.) ;
#2142=EDGE_CURVE('',#1764,#1795,#918,.F.) ;
#2143=EDGE_CURVE('',#1795,#1796,#1603,.F.) ;
#2144=EDGE_CURVE('',#1764,#1796,#919,.T.) ;
#2145=EDGE_CURVE('',#1796,#1797,#920,.F.) ;
#2146=EDGE_CURVE('',#1765,#1797,#921,.F.) ;
#2147=EDGE_CURVE('',#1797,#1798,#1604,.T.) ;
#2148=EDGE_CURVE('',#1766,#1798,#922,.F.) ;
#2149=EDGE_CURVE('',#1799,#1743,#923,.T.) ;
#2150=EDGE_CURVE('',#1798,#1799,#924,.F.) ;
#2151=EDGE_CURVE('',#1800,#1767,#925,.T.) ;
#2152=EDGE_CURVE('',#1744,#1800,#926,.F.) ;
#2153=EDGE_CURVE('',#1801,#1802,#927,.F.) ;
#2154=EDGE_CURVE('',#1803,#1801,#1605,.T.) ;
#2155=EDGE_CURVE('',#1804,#1803,#928,.F.) ;
#2156=EDGE_CURVE('',#1805,#1804,#929,.F.) ;
#2157=EDGE_CURVE('',#1806,#1805,#930,.T.) ;
#2158=EDGE_CURVE('',#1807,#1806,#931,.F.) ;
#2159=EDGE_CURVE('',#1808,#1807,#932,.T.) ;
#2160=EDGE_CURVE('',#1809,#1808,#1606,.T.) ;
#2161=EDGE_CURVE('',#1810,#1809,#933,.F.) ;
#2162=EDGE_CURVE('',#1811,#1810,#1607,.T.) ;
#2163=EDGE_CURVE('',#1812,#1811,#934,.T.) ;
#2164=EDGE_CURVE('',#1813,#1812,#935,.F.) ;
#2165=EDGE_CURVE('',#1814,#1813,#936,.F.) ;
#2166=EDGE_CURVE('',#1815,#1814,#1608,.T.) ;
#2167=EDGE_CURVE('',#1816,#1815,#937,.F.) ;
#2168=EDGE_CURVE('',#1817,#1816,#1609,.T.) ;
#2169=EDGE_CURVE('',#1818,#1817,#938,.F.) ;
#2170=EDGE_CURVE('',#1819,#1818,#939,.F.) ;
#2171=EDGE_CURVE('',#1820,#1819,#940,.F.) ;
#2172=EDGE_CURVE('',#1821,#1820,#941,.T.) ;
#2173=EDGE_CURVE('',#1822,#1821,#942,.T.) ;
#2174=EDGE_CURVE('',#1823,#1822,#1610,.T.) ;
#2175=EDGE_CURVE('',#1824,#1823,#943,.T.) ;
#2176=EDGE_CURVE('',#1727,#1824,#944,.F.) ;
#2177=EDGE_CURVE('',#1802,#1728,#945,.T.) ;
#2178=EDGE_CURVE('',#1825,#1826,#1611,.F.) ;
#2179=EDGE_CURVE('',#1778,#1826,#946,.F.) ;
#2180=EDGE_CURVE('',#1777,#1825,#947,.F.) ;
#2181=EDGE_CURVE('',#1827,#1828,#1612,.F.) ;
#2182=EDGE_CURVE('',#1780,#1828,#948,.F.) ;
#2183=EDGE_CURVE('',#1779,#1827,#949,.F.) ;
#2184=EDGE_CURVE('',#1829,#1830,#1613,.F.) ;
#2185=EDGE_CURVE('',#1786,#1830,#950,.F.) ;
#2186=EDGE_CURVE('',#1785,#1829,#951,.F.) ;
#2187=EDGE_CURVE('',#1831,#1832,#1614,.F.) ;
#2188=EDGE_CURVE('',#1788,#1832,#952,.F.) ;
#2189=EDGE_CURVE('',#1787,#1831,#953,.F.) ;
#2190=EDGE_CURVE('',#1833,#1834,#1615,.F.) ;
#2191=EDGE_CURVE('',#1798,#1834,#954,.F.) ;
#2192=EDGE_CURVE('',#1797,#1833,#955,.F.) ;
#2193=EDGE_CURVE('',#1835,#1836,#1616,.F.) ;
#2194=EDGE_CURVE('',#1768,#1836,#956,.F.) ;
#2195=EDGE_CURVE('',#1767,#1835,#957,.F.) ;
#2196=EDGE_CURVE('',#1837,#1835,#958,.T.) ;
#2197=EDGE_CURVE('',#1837,#1800,#959,.T.) ;
#2198=EDGE_CURVE('',#1830,#1831,#960,.F.) ;
#2199=EDGE_CURVE('',#1826,#1827,#961,.F.) ;
#2200=EDGE_CURVE('',#1838,#1799,#962,.T.) ;
#2201=EDGE_CURVE('',#1834,#1838,#963,.F.) ;
#2202=EDGE_CURVE('',#1837,#1824,#964,.T.) ;
#2203=EDGE_CURVE('',#1802,#1838,#965,.F.) ;
#2204=EDGE_CURVE('',#1839,#1772,#966,.T.) ;
#2205=EDGE_CURVE('',#1840,#1771,#967,.T.) ;
#2206=EDGE_CURVE('',#1840,#1839,#1617,.T.) ;
#2207=EDGE_CURVE('',#1841,#1773,#968,.T.) ;
#2208=EDGE_CURVE('',#1839,#1841,#969,.F.) ;
#2209=EDGE_CURVE('',#1842,#1774,#970,.T.) ;
#2210=EDGE_CURVE('',#1841,#1842,#1618,.T.) ;
#2211=EDGE_CURVE('',#1843,#1776,#971,.T.) ;
#2212=EDGE_CURVE('',#1843,#1825,#972,.F.) ;
#2213=EDGE_CURVE('',#1844,#1775,#973,.T.) ;
#2214=EDGE_CURVE('',#1842,#1844,#974,.F.) ;
#2215=EDGE_CURVE('',#1844,#1843,#1619,.T.) ;
#2216=EDGE_CURVE('',#1845,#1781,#975,.T.) ;
#2217=EDGE_CURVE('',#1828,#1845,#976,.F.) ;
#2218=EDGE_CURVE('',#1846,#1782,#977,.T.) ;
#2219=EDGE_CURVE('',#1845,#1846,#1620,.T.) ;
#2220=EDGE_CURVE('',#1847,#1829,#978,.T.) ;
#2221=EDGE_CURVE('',#1847,#1784,#979,.T.) ;
#2222=EDGE_CURVE('',#1848,#1783,#980,.T.) ;
#2223=EDGE_CURVE('',#1846,#1848,#981,.F.) ;
#2224=EDGE_CURVE('',#1848,#1847,#1621,.T.) ;
#2225=EDGE_CURVE('',#1832,#1849,#982,.T.) ;
#2226=EDGE_CURVE('',#1849,#1789,#983,.T.) ;
#2227=EDGE_CURVE('',#1850,#1790,#984,.T.) ;
#2228=EDGE_CURVE('',#1849,#1850,#1622,.T.) ;
#2229=EDGE_CURVE('',#1851,#1791,#985,.T.) ;
#2230=EDGE_CURVE('',#1850,#1851,#986,.F.) ;
#2231=EDGE_CURVE('',#1852,#1792,#987,.T.) ;
#2232=EDGE_CURVE('',#1851,#1852,#1623,.T.) ;
#2233=EDGE_CURVE('',#1852,#1853,#988,.T.) ;
#2234=EDGE_CURVE('',#1853,#1793,#989,.T.) ;
#2235=EDGE_CURVE('',#1854,#1794,#990,.T.) ;
#2236=EDGE_CURVE('',#1853,#1854,#1624,.T.) ;
#2237=EDGE_CURVE('',#1836,#1855,#991,.T.) ;
#2238=EDGE_CURVE('',#1855,#1769,#992,.T.) ;
#2239=EDGE_CURVE('',#1856,#1840,#993,.T.) ;
#2240=EDGE_CURVE('',#1856,#1770,#994,.T.) ;
#2241=EDGE_CURVE('',#1855,#1856,#1625,.T.) ;
#2242=EDGE_CURVE('',#1857,#1796,#995,.T.) ;
#2243=EDGE_CURVE('',#1857,#1833,#996,.F.) ;
#2244=EDGE_CURVE('',#1858,#1795,#997,.T.) ;
#2245=EDGE_CURVE('',#1854,#1858,#998,.F.) ;
#2246=EDGE_CURVE('',#1858,#1857,#1626,.T.) ;
#2247=EDGE_CURVE('',#1835,#1823,#999,.T.) ;
#2248=EDGE_CURVE('',#1836,#1822,#1000,.T.) ;
#2249=EDGE_CURVE('',#1855,#1821,#1001,.T.) ;
#2250=EDGE_CURVE('',#1856,#1821,#1002,.F.) ;
#2251=EDGE_CURVE('',#1840,#1820,#1003,.T.) ;
#2252=EDGE_CURVE('',#1839,#1820,#1004,.F.) ;
#2253=EDGE_CURVE('',#1841,#1819,#1005,.T.) ;
#2254=EDGE_CURVE('',#1842,#1819,#1006,.F.) ;
#2255=EDGE_CURVE('',#1844,#1818,#1007,.T.) ;
#2256=EDGE_CURVE('',#1843,#1818,#1008,.F.) ;
#2257=EDGE_CURVE('',#1825,#1817,#1009,.T.) ;
#2258=EDGE_CURVE('',#1826,#1816,#1010,.T.) ;
#2259=EDGE_CURVE('',#1827,#1815,#1011,.T.) ;
#2260=EDGE_CURVE('',#1828,#1814,#1012,.T.) ;
#2261=EDGE_CURVE('',#1845,#1813,#1013,.T.) ;
#2262=EDGE_CURVE('',#1846,#1813,#1014,.F.) ;
#2263=EDGE_CURVE('',#1848,#1812,#1015,.T.) ;
#2264=EDGE_CURVE('',#1847,#1812,#1016,.F.) ;
#2265=EDGE_CURVE('',#1829,#1811,#1017,.T.) ;
#2266=EDGE_CURVE('',#1830,#1810,#1018,.T.) ;
#2267=EDGE_CURVE('',#1831,#1809,#1019,.T.) ;
#2268=EDGE_CURVE('',#1832,#1808,#1020,.T.) ;
#2269=EDGE_CURVE('',#1849,#1807,#1021,.T.) ;
#2270=EDGE_CURVE('',#1850,#1807,#1022,.F.) ;
#2271=EDGE_CURVE('',#1851,#1806,#1023,.T.) ;
#2272=EDGE_CURVE('',#1852,#1806,#1024,.F.) ;
#2273=EDGE_CURVE('',#1853,#1805,#1025,.T.) ;
#2274=EDGE_CURVE('',#1854,#1805,#1026,.F.) ;
#2275=EDGE_CURVE('',#1858,#1804,#1027,.T.) ;
#2276=EDGE_CURVE('',#1857,#1804,#1028,.F.) ;
#2277=EDGE_CURVE('',#1833,#1803,#1029,.T.) ;
#2278=EDGE_CURVE('',#1834,#1801,#1030,.T.) ;
#2555=ORIENTED_EDGE('',*,*,#2031,.T.) ;
#2556=ORIENTED_EDGE('',*,*,#2032,.T.) ;
#2557=ORIENTED_EDGE('',*,*,#2033,.F.) ;
#2558=ORIENTED_EDGE('',*,*,#2034,.F.) ;
#2559=ORIENTED_EDGE('',*,*,#2035,.T.) ;
#2560=ORIENTED_EDGE('',*,*,#2031,.F.) ;
#2561=ORIENTED_EDGE('',*,*,#2036,.T.) ;
#2562=ORIENTED_EDGE('',*,*,#2037,.T.) ;
#2563=ORIENTED_EDGE('',*,*,#2038,.F.) ;
#2564=ORIENTED_EDGE('',*,*,#2039,.T.) ;
#2565=ORIENTED_EDGE('',*,*,#2033,.T.) ;
#2566=ORIENTED_EDGE('',*,*,#2040,.T.) ;
#2567=ORIENTED_EDGE('',*,*,#2041,.T.) ;
#2568=ORIENTED_EDGE('',*,*,#2042,.T.) ;
#2569=ORIENTED_EDGE('',*,*,#2043,.T.) ;
#2570=ORIENTED_EDGE('',*,*,#2042,.F.) ;
#2571=ORIENTED_EDGE('',*,*,#2043,.F.) ;
#2572=ORIENTED_EDGE('',*,*,#2044,.T.) ;
#2573=ORIENTED_EDGE('',*,*,#2045,.T.) ;
#2574=ORIENTED_EDGE('',*,*,#2044,.F.) ;
#2575=ORIENTED_EDGE('',*,*,#2046,.T.) ;
#2576=ORIENTED_EDGE('',*,*,#2047,.T.) ;
#2577=ORIENTED_EDGE('',*,*,#2048,.T.) ;
#2578=ORIENTED_EDGE('',*,*,#2047,.F.) ;
#2579=ORIENTED_EDGE('',*,*,#2048,.F.) ;
#2580=ORIENTED_EDGE('',*,*,#2049,.T.) ;
#2581=ORIENTED_EDGE('',*,*,#2050,.T.) ;
#2582=ORIENTED_EDGE('',*,*,#2049,.F.) ;
#2583=ORIENTED_EDGE('',*,*,#2051,.T.) ;
#2584=ORIENTED_EDGE('',*,*,#2052,.T.) ;
#2585=ORIENTED_EDGE('',*,*,#2053,.T.) ;
#2586=ORIENTED_EDGE('',*,*,#2052,.F.) ;
#2587=ORIENTED_EDGE('',*,*,#2053,.F.) ;
#2588=ORIENTED_EDGE('',*,*,#2054,.T.) ;
#2589=ORIENTED_EDGE('',*,*,#2055,.T.) ;
#2590=ORIENTED_EDGE('',*,*,#2054,.F.) ;
#2591=ORIENTED_EDGE('',*,*,#2056,.T.) ;
#2592=ORIENTED_EDGE('',*,*,#2057,.T.) ;
#2593=ORIENTED_EDGE('',*,*,#2058,.T.) ;
#2594=ORIENTED_EDGE('',*,*,#2057,.F.) ;
#2595=ORIENTED_EDGE('',*,*,#2058,.F.) ;
#2596=ORIENTED_EDGE('',*,*,#2059,.T.) ;
#2597=ORIENTED_EDGE('',*,*,#2060,.T.) ;
#2598=ORIENTED_EDGE('',*,*,#2059,.F.) ;
#2599=ORIENTED_EDGE('',*,*,#2061,.T.) ;
#2600=ORIENTED_EDGE('',*,*,#2038,.T.) ;
#2601=ORIENTED_EDGE('',*,*,#2062,.T.) ;
#2602=ORIENTED_EDGE('',*,*,#2063,.T.) ;
#2603=ORIENTED_EDGE('',*,*,#2064,.T.) ;
#2604=ORIENTED_EDGE('',*,*,#2065,.T.) ;
#2605=ORIENTED_EDGE('',*,*,#2066,.T.) ;
#2606=ORIENTED_EDGE('',*,*,#2067,.T.) ;
#2607=ORIENTED_EDGE('',*,*,#2068,.T.) ;
#2608=ORIENTED_EDGE('',*,*,#2069,.T.) ;
#2609=ORIENTED_EDGE('',*,*,#2070,.T.) ;
#2610=ORIENTED_EDGE('',*,*,#2071,.T.) ;
#2611=ORIENTED_EDGE('',*,*,#2072,.T.) ;
#2612=ORIENTED_EDGE('',*,*,#2073,.T.) ;
#2613=ORIENTED_EDGE('',*,*,#2074,.T.) ;
#2614=ORIENTED_EDGE('',*,*,#2075,.T.) ;
#2615=ORIENTED_EDGE('',*,*,#2076,.T.) ;
#2616=ORIENTED_EDGE('',*,*,#2077,.T.) ;
#2617=ORIENTED_EDGE('',*,*,#2078,.T.) ;
#2618=ORIENTED_EDGE('',*,*,#2079,.T.) ;
#2619=ORIENTED_EDGE('',*,*,#2080,.T.) ;
#2620=ORIENTED_EDGE('',*,*,#2081,.T.) ;
#2621=ORIENTED_EDGE('',*,*,#2082,.T.) ;
#2622=ORIENTED_EDGE('',*,*,#2083,.T.) ;
#2623=ORIENTED_EDGE('',*,*,#2084,.T.) ;
#2624=ORIENTED_EDGE('',*,*,#2085,.T.) ;
#2625=ORIENTED_EDGE('',*,*,#2086,.T.) ;
#2626=ORIENTED_EDGE('',*,*,#2087,.T.) ;
#2627=ORIENTED_EDGE('',*,*,#2088,.F.) ;
#2628=ORIENTED_EDGE('',*,*,#2064,.F.) ;
#2629=ORIENTED_EDGE('',*,*,#2088,.T.) ;
#2630=ORIENTED_EDGE('',*,*,#2089,.T.) ;
#2631=ORIENTED_EDGE('',*,*,#2090,.F.) ;
#2632=ORIENTED_EDGE('',*,*,#2065,.F.) ;
#2633=ORIENTED_EDGE('',*,*,#2090,.T.) ;
#2634=ORIENTED_EDGE('',*,*,#2091,.T.) ;
#2635=ORIENTED_EDGE('',*,*,#2092,.F.) ;
#2636=ORIENTED_EDGE('',*,*,#2092,.T.) ;
#2637=ORIENTED_EDGE('',*,*,#2093,.T.) ;
#2638=ORIENTED_EDGE('',*,*,#2094,.F.) ;
#2639=ORIENTED_EDGE('',*,*,#2066,.F.) ;
#2640=ORIENTED_EDGE('',*,*,#2094,.T.) ;
#2641=ORIENTED_EDGE('',*,*,#2095,.T.) ;
#2642=ORIENTED_EDGE('',*,*,#2096,.F.) ;
#2643=ORIENTED_EDGE('',*,*,#2096,.T.) ;
#2644=ORIENTED_EDGE('',*,*,#2097,.T.) ;
#2645=ORIENTED_EDGE('',*,*,#2098,.F.) ;
#2646=ORIENTED_EDGE('',*,*,#2067,.F.) ;
#2647=ORIENTED_EDGE('',*,*,#2098,.T.) ;
#2648=ORIENTED_EDGE('',*,*,#2099,.T.) ;
#2649=ORIENTED_EDGE('',*,*,#2100,.F.) ;
#2650=ORIENTED_EDGE('',*,*,#2100,.T.) ;
#2651=ORIENTED_EDGE('',*,*,#2101,.T.) ;
#2652=ORIENTED_EDGE('',*,*,#2102,.F.) ;
#2653=ORIENTED_EDGE('',*,*,#2068,.F.) ;
#2654=ORIENTED_EDGE('',*,*,#2102,.T.) ;
#2655=ORIENTED_EDGE('',*,*,#2103,.T.) ;
#2656=ORIENTED_EDGE('',*,*,#2104,.F.) ;
#2657=ORIENTED_EDGE('',*,*,#2104,.T.) ;
#2658=ORIENTED_EDGE('',*,*,#2105,.T.) ;
#2659=ORIENTED_EDGE('',*,*,#2106,.F.) ;
#2660=ORIENTED_EDGE('',*,*,#2069,.F.) ;
#2661=ORIENTED_EDGE('',*,*,#2106,.T.) ;
#2662=ORIENTED_EDGE('',*,*,#2107,.T.) ;
#2663=ORIENTED_EDGE('',*,*,#2108,.F.) ;
#2664=ORIENTED_EDGE('',*,*,#2070,.F.) ;
#2665=ORIENTED_EDGE('',*,*,#2108,.T.) ;
#2666=ORIENTED_EDGE('',*,*,#2109,.T.) ;
#2667=ORIENTED_EDGE('',*,*,#2110,.F.) ;
#2668=ORIENTED_EDGE('',*,*,#2071,.F.) ;
#2669=ORIENTED_EDGE('',*,*,#2110,.T.) ;
#2670=ORIENTED_EDGE('',*,*,#2111,.T.) ;
#2671=ORIENTED_EDGE('',*,*,#2112,.F.) ;
#2672=ORIENTED_EDGE('',*,*,#2072,.F.) ;
#2673=ORIENTED_EDGE('',*,*,#2112,.T.) ;
#2674=ORIENTED_EDGE('',*,*,#2113,.T.) ;
#2675=ORIENTED_EDGE('',*,*,#2114,.F.) ;
#2676=ORIENTED_EDGE('',*,*,#2073,.F.) ;
#2677=ORIENTED_EDGE('',*,*,#2114,.T.) ;
#2678=ORIENTED_EDGE('',*,*,#2115,.T.) ;
#2679=ORIENTED_EDGE('',*,*,#2116,.F.) ;
#2680=ORIENTED_EDGE('',*,*,#2116,.T.) ;
#2681=ORIENTED_EDGE('',*,*,#2117,.T.) ;
#2682=ORIENTED_EDGE('',*,*,#2118,.F.) ;
#2683=ORIENTED_EDGE('',*,*,#2074,.F.) ;
#2684=ORIENTED_EDGE('',*,*,#2118,.T.) ;
#2685=ORIENTED_EDGE('',*,*,#2119,.T.) ;
#2686=ORIENTED_EDGE('',*,*,#2120,.F.) ;
#2687=ORIENTED_EDGE('',*,*,#2120,.T.) ;
#2688=ORIENTED_EDGE('',*,*,#2121,.T.) ;
#2689=ORIENTED_EDGE('',*,*,#2122,.F.) ;
#2690=ORIENTED_EDGE('',*,*,#2075,.F.) ;
#2691=ORIENTED_EDGE('',*,*,#2122,.T.) ;
#2692=ORIENTED_EDGE('',*,*,#2123,.T.) ;
#2693=ORIENTED_EDGE('',*,*,#2124,.F.) ;
#2694=ORIENTED_EDGE('',*,*,#2076,.F.) ;
#2695=ORIENTED_EDGE('',*,*,#2124,.T.) ;
#2696=ORIENTED_EDGE('',*,*,#2125,.T.) ;
#2697=ORIENTED_EDGE('',*,*,#2126,.F.) ;
#2698=ORIENTED_EDGE('',*,*,#2077,.F.) ;
#2699=ORIENTED_EDGE('',*,*,#2126,.T.) ;
#2700=ORIENTED_EDGE('',*,*,#2127,.T.) ;
#2701=ORIENTED_EDGE('',*,*,#2128,.F.) ;
#2702=ORIENTED_EDGE('',*,*,#2078,.F.) ;
#2703=ORIENTED_EDGE('',*,*,#2128,.T.) ;
#2704=ORIENTED_EDGE('',*,*,#2129,.T.) ;
#2705=ORIENTED_EDGE('',*,*,#2130,.F.) ;
#2706=ORIENTED_EDGE('',*,*,#2079,.F.) ;
#2707=ORIENTED_EDGE('',*,*,#2130,.T.) ;
#2708=ORIENTED_EDGE('',*,*,#2131,.T.) ;
#2709=ORIENTED_EDGE('',*,*,#2132,.F.) ;
#2710=ORIENTED_EDGE('',*,*,#2132,.T.) ;
#2711=ORIENTED_EDGE('',*,*,#2133,.T.) ;
#2712=ORIENTED_EDGE('',*,*,#2134,.F.) ;
#2713=ORIENTED_EDGE('',*,*,#2080,.F.) ;
#2714=ORIENTED_EDGE('',*,*,#2134,.T.) ;
#2715=ORIENTED_EDGE('',*,*,#2135,.T.) ;
#2716=ORIENTED_EDGE('',*,*,#2136,.F.) ;
#2717=ORIENTED_EDGE('',*,*,#2136,.T.) ;
#2718=ORIENTED_EDGE('',*,*,#2137,.T.) ;
#2719=ORIENTED_EDGE('',*,*,#2138,.F.) ;
#2720=ORIENTED_EDGE('',*,*,#2081,.F.) ;
#2721=ORIENTED_EDGE('',*,*,#2138,.T.) ;
#2722=ORIENTED_EDGE('',*,*,#2139,.T.) ;
#2723=ORIENTED_EDGE('',*,*,#2140,.F.) ;
#2724=ORIENTED_EDGE('',*,*,#2140,.T.) ;
#2725=ORIENTED_EDGE('',*,*,#2141,.T.) ;
#2726=ORIENTED_EDGE('',*,*,#2142,.F.) ;
#2727=ORIENTED_EDGE('',*,*,#2082,.F.) ;
#2728=ORIENTED_EDGE('',*,*,#2142,.T.) ;
#2729=ORIENTED_EDGE('',*,*,#2143,.T.) ;
#2730=ORIENTED_EDGE('',*,*,#2144,.F.) ;
#2731=ORIENTED_EDGE('',*,*,#2144,.T.) ;
#2732=ORIENTED_EDGE('',*,*,#2145,.T.) ;
#2733=ORIENTED_EDGE('',*,*,#2146,.F.) ;
#2734=ORIENTED_EDGE('',*,*,#2083,.F.) ;
#2735=ORIENTED_EDGE('',*,*,#2146,.T.) ;
#2736=ORIENTED_EDGE('',*,*,#2147,.T.) ;
#2737=ORIENTED_EDGE('',*,*,#2148,.F.) ;
#2738=ORIENTED_EDGE('',*,*,#2084,.F.) ;
#2739=ORIENTED_EDGE('',*,*,#2149,.T.) ;
#2740=ORIENTED_EDGE('',*,*,#2085,.F.) ;
#2741=ORIENTED_EDGE('',*,*,#2148,.T.) ;
#2742=ORIENTED_EDGE('',*,*,#2150,.T.) ;
#2743=ORIENTED_EDGE('',*,*,#2151,.T.) ;
#2744=ORIENTED_EDGE('',*,*,#2086,.F.) ;
#2745=ORIENTED_EDGE('',*,*,#2063,.F.) ;
#2746=ORIENTED_EDGE('',*,*,#2152,.T.) ;
#2747=ORIENTED_EDGE('',*,*,#2153,.F.) ;
#2748=ORIENTED_EDGE('',*,*,#2154,.F.) ;
#2749=ORIENTED_EDGE('',*,*,#2155,.F.) ;
#2750=ORIENTED_EDGE('',*,*,#2156,.F.) ;
#2751=ORIENTED_EDGE('',*,*,#2157,.F.) ;
#2752=ORIENTED_EDGE('',*,*,#2158,.F.) ;
#2753=ORIENTED_EDGE('',*,*,#2159,.F.) ;
#2754=ORIENTED_EDGE('',*,*,#2160,.F.) ;
#2755=ORIENTED_EDGE('',*,*,#2161,.F.) ;
#2756=ORIENTED_EDGE('',*,*,#2162,.F.) ;
#2757=ORIENTED_EDGE('',*,*,#2163,.F.) ;
#2758=ORIENTED_EDGE('',*,*,#2164,.F.) ;
#2759=ORIENTED_EDGE('',*,*,#2165,.F.) ;
#2760=ORIENTED_EDGE('',*,*,#2166,.F.) ;
#2761=ORIENTED_EDGE('',*,*,#2167,.F.) ;
#2762=ORIENTED_EDGE('',*,*,#2168,.F.) ;
#2763=ORIENTED_EDGE('',*,*,#2169,.F.) ;
#2764=ORIENTED_EDGE('',*,*,#2170,.F.) ;
#2765=ORIENTED_EDGE('',*,*,#2171,.F.) ;
#2766=ORIENTED_EDGE('',*,*,#2172,.F.) ;
#2767=ORIENTED_EDGE('',*,*,#2173,.F.) ;
#2768=ORIENTED_EDGE('',*,*,#2174,.F.) ;
#2769=ORIENTED_EDGE('',*,*,#2175,.F.) ;
#2770=ORIENTED_EDGE('',*,*,#2176,.F.) ;
#2771=ORIENTED_EDGE('',*,*,#2037,.F.) ;
#2772=ORIENTED_EDGE('',*,*,#2177,.F.) ;
#2773=ORIENTED_EDGE('',*,*,#2178,.T.) ;
#2774=ORIENTED_EDGE('',*,*,#2179,.F.) ;
#2775=ORIENTED_EDGE('',*,*,#2107,.F.) ;
#2776=ORIENTED_EDGE('',*,*,#2180,.T.) ;
#2777=ORIENTED_EDGE('',*,*,#2181,.T.) ;
#2778=ORIENTED_EDGE('',*,*,#2182,.F.) ;
#2779=ORIENTED_EDGE('',*,*,#2111,.F.) ;
#2780=ORIENTED_EDGE('',*,*,#2183,.T.) ;
#2781=ORIENTED_EDGE('',*,*,#2184,.T.) ;
#2782=ORIENTED_EDGE('',*,*,#2185,.F.) ;
#2783=ORIENTED_EDGE('',*,*,#2123,.F.) ;
#2784=ORIENTED_EDGE('',*,*,#2186,.T.) ;
#2785=ORIENTED_EDGE('',*,*,#2187,.T.) ;
#2786=ORIENTED_EDGE('',*,*,#2188,.F.) ;
#2787=ORIENTED_EDGE('',*,*,#2127,.F.) ;
#2788=ORIENTED_EDGE('',*,*,#2189,.T.) ;
#2789=ORIENTED_EDGE('',*,*,#2190,.T.) ;
#2790=ORIENTED_EDGE('',*,*,#2191,.F.) ;
#2791=ORIENTED_EDGE('',*,*,#2147,.F.) ;
#2792=ORIENTED_EDGE('',*,*,#2192,.T.) ;
#2793=ORIENTED_EDGE('',*,*,#2193,.T.) ;
#2794=ORIENTED_EDGE('',*,*,#2194,.F.) ;
#2795=ORIENTED_EDGE('',*,*,#2087,.F.) ;
#2796=ORIENTED_EDGE('',*,*,#2195,.T.) ;
#2797=ORIENTED_EDGE('',*,*,#2196,.T.) ;
#2798=ORIENTED_EDGE('',*,*,#2195,.F.) ;
#2799=ORIENTED_EDGE('',*,*,#2151,.F.) ;
#2800=ORIENTED_EDGE('',*,*,#2197,.F.) ;
#2801=ORIENTED_EDGE('',*,*,#2189,.F.) ;
#2802=ORIENTED_EDGE('',*,*,#2125,.F.) ;
#2803=ORIENTED_EDGE('',*,*,#2185,.T.) ;
#2804=ORIENTED_EDGE('',*,*,#2198,.T.) ;
#2805=ORIENTED_EDGE('',*,*,#2183,.F.) ;
#2806=ORIENTED_EDGE('',*,*,#2109,.F.) ;
#2807=ORIENTED_EDGE('',*,*,#2179,.T.) ;
#2808=ORIENTED_EDGE('',*,*,#2199,.T.) ;
#2809=ORIENTED_EDGE('',*,*,#2200,.T.) ;
#2810=ORIENTED_EDGE('',*,*,#2150,.F.) ;
#2811=ORIENTED_EDGE('',*,*,#2191,.T.) ;
#2812=ORIENTED_EDGE('',*,*,#2201,.T.) ;
#2813=ORIENTED_EDGE('',*,*,#2197,.T.) ;
#2814=ORIENTED_EDGE('',*,*,#2152,.F.) ;
#2815=ORIENTED_EDGE('',*,*,#2062,.F.) ;
#2816=ORIENTED_EDGE('',*,*,#2040,.F.) ;
#2817=ORIENTED_EDGE('',*,*,#2032,.F.) ;
#2818=ORIENTED_EDGE('',*,*,#2035,.F.) ;
#2819=ORIENTED_EDGE('',*,*,#2176,.T.) ;
#2820=ORIENTED_EDGE('',*,*,#2202,.F.) ;
#2821=ORIENTED_EDGE('',*,*,#2041,.F.) ;
#2822=ORIENTED_EDGE('',*,*,#2046,.F.) ;
#2823=ORIENTED_EDGE('',*,*,#2177,.T.) ;
#2824=ORIENTED_EDGE('',*,*,#2036,.F.) ;
#2825=ORIENTED_EDGE('',*,*,#2034,.T.) ;
#2826=ORIENTED_EDGE('',*,*,#2039,.F.) ;
#2827=ORIENTED_EDGE('',*,*,#2061,.F.) ;
#2828=ORIENTED_EDGE('',*,*,#2149,.F.) ;
#2829=ORIENTED_EDGE('',*,*,#2200,.F.) ;
#2830=ORIENTED_EDGE('',*,*,#2203,.F.) ;
#2831=ORIENTED_EDGE('',*,*,#2056,.F.) ;
#2832=ORIENTED_EDGE('',*,*,#2051,.F.) ;
#2833=ORIENTED_EDGE('',*,*,#2204,.T.) ;
#2834=ORIENTED_EDGE('',*,*,#2095,.F.) ;
#2835=ORIENTED_EDGE('',*,*,#2205,.F.) ;
#2836=ORIENTED_EDGE('',*,*,#2206,.T.) ;
#2837=ORIENTED_EDGE('',*,*,#2207,.T.) ;
#2838=ORIENTED_EDGE('',*,*,#2097,.F.) ;
#2839=ORIENTED_EDGE('',*,*,#2204,.F.) ;
#2840=ORIENTED_EDGE('',*,*,#2208,.T.) ;
#2841=ORIENTED_EDGE('',*,*,#2209,.T.) ;
#2842=ORIENTED_EDGE('',*,*,#2099,.F.) ;
#2843=ORIENTED_EDGE('',*,*,#2207,.F.) ;
#2844=ORIENTED_EDGE('',*,*,#2210,.T.) ;
#2845=ORIENTED_EDGE('',*,*,#2180,.F.) ;
#2846=ORIENTED_EDGE('',*,*,#2105,.F.) ;
#2847=ORIENTED_EDGE('',*,*,#2211,.F.) ;
#2848=ORIENTED_EDGE('',*,*,#2212,.T.) ;
#2849=ORIENTED_EDGE('',*,*,#2213,.T.) ;
#2850=ORIENTED_EDGE('',*,*,#2101,.F.) ;
#2851=ORIENTED_EDGE('',*,*,#2209,.F.) ;
#2852=ORIENTED_EDGE('',*,*,#2214,.T.) ;
#2853=ORIENTED_EDGE('',*,*,#2050,.F.) ;
#2854=ORIENTED_EDGE('',*,*,#2045,.F.) ;
#2855=ORIENTED_EDGE('',*,*,#2211,.T.) ;
#2856=ORIENTED_EDGE('',*,*,#2103,.F.) ;
#2857=ORIENTED_EDGE('',*,*,#2213,.F.) ;
#2858=ORIENTED_EDGE('',*,*,#2215,.T.) ;
#2859=ORIENTED_EDGE('',*,*,#2216,.T.) ;
#2860=ORIENTED_EDGE('',*,*,#2113,.F.) ;
#2861=ORIENTED_EDGE('',*,*,#2182,.T.) ;
#2862=ORIENTED_EDGE('',*,*,#2217,.T.) ;
#2863=ORIENTED_EDGE('',*,*,#2218,.T.) ;
#2864=ORIENTED_EDGE('',*,*,#2115,.F.) ;
#2865=ORIENTED_EDGE('',*,*,#2216,.F.) ;
#2866=ORIENTED_EDGE('',*,*,#2219,.T.) ;
#2867=ORIENTED_EDGE('',*,*,#2220,.T.) ;
#2868=ORIENTED_EDGE('',*,*,#2186,.F.) ;
#2869=ORIENTED_EDGE('',*,*,#2121,.F.) ;
#2870=ORIENTED_EDGE('',*,*,#2221,.F.) ;
#2871=ORIENTED_EDGE('',*,*,#2222,.T.) ;
#2872=ORIENTED_EDGE('',*,*,#2117,.F.) ;
#2873=ORIENTED_EDGE('',*,*,#2218,.F.) ;
#2874=ORIENTED_EDGE('',*,*,#2223,.T.) ;
#2875=ORIENTED_EDGE('',*,*,#2221,.T.) ;
#2876=ORIENTED_EDGE('',*,*,#2119,.F.) ;
#2877=ORIENTED_EDGE('',*,*,#2222,.F.) ;
#2878=ORIENTED_EDGE('',*,*,#2224,.T.) ;
#2879=ORIENTED_EDGE('',*,*,#2225,.T.) ;
#2880=ORIENTED_EDGE('',*,*,#2226,.T.) ;
#2881=ORIENTED_EDGE('',*,*,#2129,.F.) ;
#2882=ORIENTED_EDGE('',*,*,#2188,.T.) ;
#2883=ORIENTED_EDGE('',*,*,#2227,.T.) ;
#2884=ORIENTED_EDGE('',*,*,#2131,.F.) ;
#2885=ORIENTED_EDGE('',*,*,#2226,.F.) ;
#2886=ORIENTED_EDGE('',*,*,#2228,.T.) ;
#2887=ORIENTED_EDGE('',*,*,#2229,.T.) ;
#2888=ORIENTED_EDGE('',*,*,#2133,.F.) ;
#2889=ORIENTED_EDGE('',*,*,#2227,.F.) ;
#2890=ORIENTED_EDGE('',*,*,#2230,.T.) ;
#2891=ORIENTED_EDGE('',*,*,#2060,.F.) ;
#2892=ORIENTED_EDGE('',*,*,#2055,.F.) ;
#2893=ORIENTED_EDGE('',*,*,#2231,.T.) ;
#2894=ORIENTED_EDGE('',*,*,#2135,.F.) ;
#2895=ORIENTED_EDGE('',*,*,#2229,.F.) ;
#2896=ORIENTED_EDGE('',*,*,#2232,.T.) ;
#2897=ORIENTED_EDGE('',*,*,#2233,.T.) ;
#2898=ORIENTED_EDGE('',*,*,#2234,.T.) ;
#2899=ORIENTED_EDGE('',*,*,#2137,.F.) ;
#2900=ORIENTED_EDGE('',*,*,#2231,.F.) ;
#2901=ORIENTED_EDGE('',*,*,#2235,.T.) ;
#2902=ORIENTED_EDGE('',*,*,#2139,.F.) ;
#2903=ORIENTED_EDGE('',*,*,#2234,.F.) ;
#2904=ORIENTED_EDGE('',*,*,#2236,.T.) ;
#2905=ORIENTED_EDGE('',*,*,#2237,.T.) ;
#2906=ORIENTED_EDGE('',*,*,#2238,.T.) ;
#2907=ORIENTED_EDGE('',*,*,#2089,.F.) ;
#2908=ORIENTED_EDGE('',*,*,#2194,.T.) ;
#2909=ORIENTED_EDGE('',*,*,#2239,.T.) ;
#2910=ORIENTED_EDGE('',*,*,#2205,.T.) ;
#2911=ORIENTED_EDGE('',*,*,#2093,.F.) ;
#2912=ORIENTED_EDGE('',*,*,#2240,.F.) ;
#2913=ORIENTED_EDGE('',*,*,#2240,.T.) ;
#2914=ORIENTED_EDGE('',*,*,#2091,.F.) ;
#2915=ORIENTED_EDGE('',*,*,#2238,.F.) ;
#2916=ORIENTED_EDGE('',*,*,#2241,.T.) ;
#2917=ORIENTED_EDGE('',*,*,#2192,.F.) ;
#2918=ORIENTED_EDGE('',*,*,#2145,.F.) ;
#2919=ORIENTED_EDGE('',*,*,#2242,.F.) ;
#2920=ORIENTED_EDGE('',*,*,#2243,.T.) ;
#2921=ORIENTED_EDGE('',*,*,#2244,.T.) ;
#2922=ORIENTED_EDGE('',*,*,#2141,.F.) ;
#2923=ORIENTED_EDGE('',*,*,#2235,.F.) ;
#2924=ORIENTED_EDGE('',*,*,#2245,.T.) ;
#2925=ORIENTED_EDGE('',*,*,#2242,.T.) ;
#2926=ORIENTED_EDGE('',*,*,#2143,.F.) ;
#2927=ORIENTED_EDGE('',*,*,#2244,.F.) ;
#2928=ORIENTED_EDGE('',*,*,#2246,.T.) ;
#2929=ORIENTED_EDGE('',*,*,#2247,.T.) ;
#2930=ORIENTED_EDGE('',*,*,#2174,.T.) ;
#2931=ORIENTED_EDGE('',*,*,#2248,.F.) ;
#2932=ORIENTED_EDGE('',*,*,#2193,.F.) ;
#2933=ORIENTED_EDGE('',*,*,#2248,.T.) ;
#2934=ORIENTED_EDGE('',*,*,#2173,.T.) ;
#2935=ORIENTED_EDGE('',*,*,#2249,.F.) ;
#2936=ORIENTED_EDGE('',*,*,#2237,.F.) ;
#2937=ORIENTED_EDGE('',*,*,#2249,.T.) ;
#2938=ORIENTED_EDGE('',*,*,#2250,.F.) ;
#2939=ORIENTED_EDGE('',*,*,#2241,.F.) ;
#2940=ORIENTED_EDGE('',*,*,#2250,.T.) ;
#2941=ORIENTED_EDGE('',*,*,#2172,.T.) ;
#2942=ORIENTED_EDGE('',*,*,#2251,.F.) ;
#2943=ORIENTED_EDGE('',*,*,#2239,.F.) ;
#2944=ORIENTED_EDGE('',*,*,#2251,.T.) ;
#2945=ORIENTED_EDGE('',*,*,#2252,.F.) ;
#2946=ORIENTED_EDGE('',*,*,#2206,.F.) ;
#2947=ORIENTED_EDGE('',*,*,#2252,.T.) ;
#2948=ORIENTED_EDGE('',*,*,#2171,.T.) ;
#2949=ORIENTED_EDGE('',*,*,#2253,.F.) ;
#2950=ORIENTED_EDGE('',*,*,#2208,.F.) ;
#2951=ORIENTED_EDGE('',*,*,#2253,.T.) ;
#2952=ORIENTED_EDGE('',*,*,#2254,.F.) ;
#2953=ORIENTED_EDGE('',*,*,#2210,.F.) ;
#2954=ORIENTED_EDGE('',*,*,#2254,.T.) ;
#2955=ORIENTED_EDGE('',*,*,#2170,.T.) ;
#2956=ORIENTED_EDGE('',*,*,#2255,.F.) ;
#2957=ORIENTED_EDGE('',*,*,#2214,.F.) ;
#2958=ORIENTED_EDGE('',*,*,#2255,.T.) ;
#2959=ORIENTED_EDGE('',*,*,#2256,.F.) ;
#2960=ORIENTED_EDGE('',*,*,#2215,.F.) ;
#2961=ORIENTED_EDGE('',*,*,#2256,.T.) ;
#2962=ORIENTED_EDGE('',*,*,#2169,.T.) ;
#2963=ORIENTED_EDGE('',*,*,#2257,.F.) ;
#2964=ORIENTED_EDGE('',*,*,#2212,.F.) ;
#2965=ORIENTED_EDGE('',*,*,#2257,.T.) ;
#2966=ORIENTED_EDGE('',*,*,#2168,.T.) ;
#2967=ORIENTED_EDGE('',*,*,#2258,.F.) ;
#2968=ORIENTED_EDGE('',*,*,#2178,.F.) ;
#2969=ORIENTED_EDGE('',*,*,#2258,.T.) ;
#2970=ORIENTED_EDGE('',*,*,#2167,.T.) ;
#2971=ORIENTED_EDGE('',*,*,#2259,.F.) ;
#2972=ORIENTED_EDGE('',*,*,#2199,.F.) ;
#2973=ORIENTED_EDGE('',*,*,#2259,.T.) ;
#2974=ORIENTED_EDGE('',*,*,#2166,.T.) ;
#2975=ORIENTED_EDGE('',*,*,#2260,.F.) ;
#2976=ORIENTED_EDGE('',*,*,#2181,.F.) ;
#2977=ORIENTED_EDGE('',*,*,#2260,.T.) ;
#2978=ORIENTED_EDGE('',*,*,#2165,.T.) ;
#2979=ORIENTED_EDGE('',*,*,#2261,.F.) ;
#2980=ORIENTED_EDGE('',*,*,#2217,.F.) ;
#2981=ORIENTED_EDGE('',*,*,#2261,.T.) ;
#2982=ORIENTED_EDGE('',*,*,#2262,.F.) ;
#2983=ORIENTED_EDGE('',*,*,#2219,.F.) ;
#2984=ORIENTED_EDGE('',*,*,#2262,.T.) ;
#2985=ORIENTED_EDGE('',*,*,#2164,.T.) ;
#2986=ORIENTED_EDGE('',*,*,#2263,.F.) ;
#2987=ORIENTED_EDGE('',*,*,#2223,.F.) ;
#2988=ORIENTED_EDGE('',*,*,#2263,.T.) ;
#2989=ORIENTED_EDGE('',*,*,#2264,.F.) ;
#2990=ORIENTED_EDGE('',*,*,#2224,.F.) ;
#2991=ORIENTED_EDGE('',*,*,#2264,.T.) ;
#2992=ORIENTED_EDGE('',*,*,#2163,.T.) ;
#2993=ORIENTED_EDGE('',*,*,#2265,.F.) ;
#2994=ORIENTED_EDGE('',*,*,#2220,.F.) ;
#2995=ORIENTED_EDGE('',*,*,#2265,.T.) ;
#2996=ORIENTED_EDGE('',*,*,#2162,.T.) ;
#2997=ORIENTED_EDGE('',*,*,#2266,.F.) ;
#2998=ORIENTED_EDGE('',*,*,#2184,.F.) ;
#2999=ORIENTED_EDGE('',*,*,#2266,.T.) ;
#3000=ORIENTED_EDGE('',*,*,#2161,.T.) ;
#3001=ORIENTED_EDGE('',*,*,#2267,.F.) ;
#3002=ORIENTED_EDGE('',*,*,#2198,.F.) ;
#3003=ORIENTED_EDGE('',*,*,#2267,.T.) ;
#3004=ORIENTED_EDGE('',*,*,#2160,.T.) ;
#3005=ORIENTED_EDGE('',*,*,#2268,.F.) ;
#3006=ORIENTED_EDGE('',*,*,#2187,.F.) ;
#3007=ORIENTED_EDGE('',*,*,#2268,.T.) ;
#3008=ORIENTED_EDGE('',*,*,#2159,.T.) ;
#3009=ORIENTED_EDGE('',*,*,#2269,.F.) ;
#3010=ORIENTED_EDGE('',*,*,#2225,.F.) ;
#3011=ORIENTED_EDGE('',*,*,#2269,.T.) ;
#3012=ORIENTED_EDGE('',*,*,#2270,.F.) ;
#3013=ORIENTED_EDGE('',*,*,#2228,.F.) ;
#3014=ORIENTED_EDGE('',*,*,#2270,.T.) ;
#3015=ORIENTED_EDGE('',*,*,#2158,.T.) ;
#3016=ORIENTED_EDGE('',*,*,#2271,.F.) ;
#3017=ORIENTED_EDGE('',*,*,#2230,.F.) ;
#3018=ORIENTED_EDGE('',*,*,#2271,.T.) ;
#3019=ORIENTED_EDGE('',*,*,#2272,.F.) ;
#3020=ORIENTED_EDGE('',*,*,#2232,.F.) ;
#3021=ORIENTED_EDGE('',*,*,#2272,.T.) ;
#3022=ORIENTED_EDGE('',*,*,#2157,.T.) ;
#3023=ORIENTED_EDGE('',*,*,#2273,.F.) ;
#3024=ORIENTED_EDGE('',*,*,#2233,.F.) ;
#3025=ORIENTED_EDGE('',*,*,#2273,.T.) ;
#3026=ORIENTED_EDGE('',*,*,#2274,.F.) ;
#3027=ORIENTED_EDGE('',*,*,#2236,.F.) ;
#3028=ORIENTED_EDGE('',*,*,#2274,.T.) ;
#3029=ORIENTED_EDGE('',*,*,#2156,.T.) ;
#3030=ORIENTED_EDGE('',*,*,#2275,.F.) ;
#3031=ORIENTED_EDGE('',*,*,#2245,.F.) ;
#3032=ORIENTED_EDGE('',*,*,#2275,.T.) ;
#3033=ORIENTED_EDGE('',*,*,#2276,.F.) ;
#3034=ORIENTED_EDGE('',*,*,#2246,.F.) ;
#3035=ORIENTED_EDGE('',*,*,#2276,.T.) ;
#3036=ORIENTED_EDGE('',*,*,#2155,.T.) ;
#3037=ORIENTED_EDGE('',*,*,#2277,.F.) ;
#3038=ORIENTED_EDGE('',*,*,#2243,.F.) ;
#3039=ORIENTED_EDGE('',*,*,#2277,.T.) ;
#3040=ORIENTED_EDGE('',*,*,#2154,.T.) ;
#3041=ORIENTED_EDGE('',*,*,#2278,.F.) ;
#3042=ORIENTED_EDGE('',*,*,#2190,.F.) ;
#3043=ORIENTED_EDGE('',*,*,#2201,.F.) ;
#3044=ORIENTED_EDGE('',*,*,#2278,.T.) ;
#3045=ORIENTED_EDGE('',*,*,#2153,.T.) ;
#3046=ORIENTED_EDGE('',*,*,#2203,.T.) ;
#3047=ORIENTED_EDGE('',*,*,#2202,.T.) ;
#3048=ORIENTED_EDGE('',*,*,#2175,.T.) ;
#3049=ORIENTED_EDGE('',*,*,#2247,.F.) ;
#3050=ORIENTED_EDGE('',*,*,#2196,.F.) ;
#3603=CYLINDRICAL_SURFACE('',#4018,27.5) ;
#3604=CYLINDRICAL_SURFACE('',#4025,3.25) ;
#3605=CYLINDRICAL_SURFACE('',#4030,3.25) ;
#3606=CYLINDRICAL_SURFACE('',#4035,3.25) ;
#3607=CYLINDRICAL_SURFACE('',#4040,3.25) ;
#3608=CYLINDRICAL_SURFACE('',#4108,0.8) ;
#3609=CYLINDRICAL_SURFACE('',#4110,0.8) ;
#3610=CYLINDRICAL_SURFACE('',#4112,0.8) ;
#3611=CYLINDRICAL_SURFACE('',#4114,0.8) ;
#3612=CYLINDRICAL_SURFACE('',#4116,0.8) ;
#3613=CYLINDRICAL_SURFACE('',#4118,0.8) ;
#3614=CYLINDRICAL_SURFACE('',#4126,0.6) ;
#3615=CYLINDRICAL_SURFACE('',#4129,0.6) ;
#3616=CYLINDRICAL_SURFACE('',#4133,0.6) ;
#3617=CYLINDRICAL_SURFACE('',#4136,0.6) ;
#3618=CYLINDRICAL_SURFACE('',#4140,0.6) ;
#3619=CYLINDRICAL_SURFACE('',#4143,0.6) ;
#3620=CYLINDRICAL_SURFACE('',#4146,0.6) ;
#3621=CYLINDRICAL_SURFACE('',#4149,0.6) ;
#3622=CYLINDRICAL_SURFACE('',#4153,0.6) ;
#3623=CYLINDRICAL_SURFACE('',#4157,0.6) ;
#3651=ADVANCED_FACE('',(#327),#3603,.F.) ;
#3652=ADVANCED_FACE('',(#328),#267,.F.) ;
#3653=ADVANCED_FACE('',(#329),#268,.F.) ;
#3654=ADVANCED_FACE('',(#330),#3604,.F.) ;
#3655=ADVANCED_FACE('',(#331),#269,.F.) ;
#3656=ADVANCED_FACE('',(#332),#3605,.F.) ;
#3657=ADVANCED_FACE('',(#333),#270,.F.) ;
#3658=ADVANCED_FACE('',(#334),#3606,.F.) ;
#3659=ADVANCED_FACE('',(#335),#271,.F.) ;
#3660=ADVANCED_FACE('',(#336),#3607,.F.) ;
#3661=ADVANCED_FACE('',(#337),#272,.F.) ;
#3662=ADVANCED_FACE('',(#338),#135,.T.) ;
#3663=ADVANCED_FACE('',(#339),#273,.F.) ;
#3664=ADVANCED_FACE('',(#340),#136,.T.) ;
#3665=ADVANCED_FACE('',(#341),#274,.T.) ;
#3666=ADVANCED_FACE('',(#342),#137,.T.) ;
#3667=ADVANCED_FACE('',(#343),#275,.T.) ;
#3668=ADVANCED_FACE('',(#344),#138,.F.) ;
#3669=ADVANCED_FACE('',(#345),#276,.T.) ;
#3670=ADVANCED_FACE('',(#346),#139,.F.) ;
#3671=ADVANCED_FACE('',(#347),#277,.T.) ;
#3672=ADVANCED_FACE('',(#348),#140,.F.) ;
#3673=ADVANCED_FACE('',(#349),#278,.F.) ;
#3674=ADVANCED_FACE('',(#350),#141,.F.) ;
#3675=ADVANCED_FACE('',(#351),#279,.F.) ;
#3676=ADVANCED_FACE('',(#352),#142,.F.) ;
#3677=ADVANCED_FACE('',(#353),#280,.T.) ;
#3678=ADVANCED_FACE('',(#354),#143,.F.) ;
#3679=ADVANCED_FACE('',(#355),#281,.T.) ;
#3680=ADVANCED_FACE('',(#356),#144,.T.) ;
#3681=ADVANCED_FACE('',(#357),#282,.F.) ;
#3682=ADVANCED_FACE('',(#358),#145,.F.) ;
#3683=ADVANCED_FACE('',(#359),#283,.F.) ;
#3684=ADVANCED_FACE('',(#360),#146,.T.) ;
#3685=ADVANCED_FACE('',(#361),#284,.T.) ;
#3686=ADVANCED_FACE('',(#362),#147,.F.) ;
#3687=ADVANCED_FACE('',(#363),#285,.T.) ;
#3688=ADVANCED_FACE('',(#364),#148,.T.) ;
#3689=ADVANCED_FACE('',(#365),#286,.T.) ;
#3690=ADVANCED_FACE('',(#366),#149,.F.) ;
#3691=ADVANCED_FACE('',(#367),#287,.T.) ;
#3692=ADVANCED_FACE('',(#368),#150,.F.) ;
#3693=ADVANCED_FACE('',(#369),#288,.F.) ;
#3694=ADVANCED_FACE('',(#370),#151,.F.) ;
#3695=ADVANCED_FACE('',(#371),#152,.T.) ;
#3696=ADVANCED_FACE('',(#372),#153,.F.) ;
#3697=ADVANCED_FACE('',(#373),#3608,.F.) ;
#3698=ADVANCED_FACE('',(#374),#3609,.F.) ;
#3699=ADVANCED_FACE('',(#375),#3610,.F.) ;
#3700=ADVANCED_FACE('',(#376),#3611,.F.) ;
#3701=ADVANCED_FACE('',(#377),#3612,.F.) ;
#3702=ADVANCED_FACE('',(#378),#3613,.F.) ;
#3703=ADVANCED_FACE('',(#379),#154,.F.) ;
#3704=ADVANCED_FACE('',(#380),#155,.T.) ;
#3705=ADVANCED_FACE('',(#381),#156,.T.) ;
#3706=ADVANCED_FACE('',(#382),#157,.T.) ;
#3707=ADVANCED_FACE('',(#383,#103,#104),#158,.T.) ;
#3708=ADVANCED_FACE('',(#384,#105,#106),#159,.T.) ;
#3709=ADVANCED_FACE('',(#385),#3614,.T.) ;
#3710=ADVANCED_FACE('',(#386),#160,.T.) ;
#3711=ADVANCED_FACE('',(#387),#3615,.T.) ;
#3712=ADVANCED_FACE('',(#388),#161,.T.) ;
#3713=ADVANCED_FACE('',(#389,#107,#108),#162,.T.) ;
#3714=ADVANCED_FACE('',(#390),#3616,.T.) ;
#3715=ADVANCED_FACE('',(#391),#163,.T.) ;
#3716=ADVANCED_FACE('',(#392),#3617,.T.) ;
#3717=ADVANCED_FACE('',(#393),#164,.F.) ;
#3718=ADVANCED_FACE('',(#394),#165,.T.) ;
#3719=ADVANCED_FACE('',(#395),#3618,.T.) ;
#3720=ADVANCED_FACE('',(#396),#166,.F.) ;
#3721=ADVANCED_FACE('',(#397),#3619,.T.) ;
#3722=ADVANCED_FACE('',(#398,#109,#110),#167,.T.) ;
#3723=ADVANCED_FACE('',(#399),#3620,.T.) ;
#3724=ADVANCED_FACE('',(#400),#168,.F.) ;
#3725=ADVANCED_FACE('',(#401),#3621,.T.) ;
#3726=ADVANCED_FACE('',(#402),#169,.F.) ;
#3727=ADVANCED_FACE('',(#403),#170,.F.) ;
#3728=ADVANCED_FACE('',(#404),#3622,.T.) ;
#3729=ADVANCED_FACE('',(#405),#171,.T.) ;
#3730=ADVANCED_FACE('',(#406),#172,.T.) ;
#3731=ADVANCED_FACE('',(#407),#3623,.T.) ;
#3732=ADVANCED_FACE('',(#408),#289,.F.) ;
#3733=ADVANCED_FACE('',(#409),#173,.F.) ;
#3734=ADVANCED_FACE('',(#410),#290,.T.) ;
#3735=ADVANCED_FACE('',(#411),#174,.F.) ;
#3736=ADVANCED_FACE('',(#412),#291,.T.) ;
#3737=ADVANCED_FACE('',(#413),#175,.T.) ;
#3738=ADVANCED_FACE('',(#414),#292,.T.) ;
#3739=ADVANCED_FACE('',(#415),#176,.T.) ;
#3740=ADVANCED_FACE('',(#416),#293,.T.) ;
#3741=ADVANCED_FACE('',(#417),#177,.T.) ;
#3742=ADVANCED_FACE('',(#418),#294,.F.) ;
#3743=ADVANCED_FACE('',(#419),#178,.T.) ;
#3744=ADVANCED_FACE('',(#420),#295,.F.) ;
#3745=ADVANCED_FACE('',(#421),#179,.T.) ;
#3746=ADVANCED_FACE('',(#422),#296,.T.) ;
#3747=ADVANCED_FACE('',(#423),#180,.T.) ;
#3748=ADVANCED_FACE('',(#424),#297,.T.) ;
#3749=ADVANCED_FACE('',(#425),#181,.F.) ;
#3750=ADVANCED_FACE('',(#426),#298,.F.) ;
#3751=ADVANCED_FACE('',(#427),#182,.T.) ;
#3752=ADVANCED_FACE('',(#428),#299,.F.) ;
#3753=ADVANCED_FACE('',(#429),#183,.F.) ;
#3754=ADVANCED_FACE('',(#430),#300,.T.) ;
#3755=ADVANCED_FACE('',(#431),#184,.T.) ;
#3756=ADVANCED_FACE('',(#432),#301,.T.) ;
#3757=ADVANCED_FACE('',(#433),#185,.F.) ;
#3758=ADVANCED_FACE('',(#434),#302,.T.) ;
#3759=ADVANCED_FACE('',(#435),#186,.T.) ;
#3760=ADVANCED_FACE('',(#436),#303,.T.) ;
#3761=ADVANCED_FACE('',(#437),#187,.T.) ;
#3762=ADVANCED_FACE('',(#438),#304,.F.) ;
#3763=ADVANCED_FACE('',(#439),#188,.T.) ;
#3764=ADVANCED_FACE('',(#440),#189,.F.) ;
#3895=CLOSED_SHELL('',(#3651,#3652,#3653,#3654,#3655,#3656,#3657,#3658,
#3659,#3660,#3661,#3662,#3663,#3664,#3665,#3666,#3667,#3668,#3669,#3670,
#3671,#3672,#3673,#3674,#3675,#3676,#3677,#3678,#3679,#3680,#3681,#3682,
#3683,#3684,#3685,#3686,#3687,#3688,#3689,#3690,#3691,#3692,#3693,#3694,
#3695,#3696,#3697,#3698,#3699,#3700,#3701,#3702,#3703,#3704,#3705,#3706,
#3707,#3708,#3709,#3710,#3711,#3712,#3713,#3714,#3715,#3716,#3717,#3718,
#3719,#3720,#3721,#3722,#3723,#3724,#3725,#3726,#3727,#3728,#3729,#3730,
#3731,#3732,#3733,#3734,#3735,#3736,#3737,#3738,#3739,#3740,#3741,#3742,
#3743,#3744,#3745,#3746,#3747,#3748,#3749,#3750,#3751,#3752,#3753,#3754,
#3755,#3756,#3757,#3758,#3759,#3760,#3761,#3762,#3763,#3764)) ;
#4017=AXIS2_PLACEMENT_3D('',#5640,#4439,#4440) ;
#4018=AXIS2_PLACEMENT_3D('',#5641,#4441,#4442) ;
#4019=AXIS2_PLACEMENT_3D('',#5644,#4443,#4444) ;
#4020=AXIS2_PLACEMENT_3D('',#5648,#4446,#4447) ;
#4021=AXIS2_PLACEMENT_3D('',#5650,#4449,#4450) ;
#4022=AXIS2_PLACEMENT_3D('',#5659,#4451,#4452) ;
#4023=AXIS2_PLACEMENT_3D('',#5660,#4453,#4454) ;
#4024=AXIS2_PLACEMENT_3D('',#5663,#4455,#4456) ;
#4025=AXIS2_PLACEMENT_3D('',#5670,#4457,#4458) ;
#4026=AXIS2_PLACEMENT_3D('',#5672,#4459,#4460) ;
#4027=AXIS2_PLACEMENT_3D('',#5675,#4462,#4463) ;
#4028=AXIS2_PLACEMENT_3D('',#5676,#4464,#4465) ;
#4029=AXIS2_PLACEMENT_3D('',#5679,#4467,#4468) ;
#4030=AXIS2_PLACEMENT_3D('',#5680,#4469,#4470) ;
#4031=AXIS2_PLACEMENT_3D('',#5682,#4471,#4472) ;
#4032=AXIS2_PLACEMENT_3D('',#5685,#4474,#4475) ;
#4033=AXIS2_PLACEMENT_3D('',#5686,#4476,#4477) ;
#4034=AXIS2_PLACEMENT_3D('',#5689,#4479,#4480) ;
#4035=AXIS2_PLACEMENT_3D('',#5690,#4481,#4482) ;
#4036=AXIS2_PLACEMENT_3D('',#5692,#4483,#4484) ;
#4037=AXIS2_PLACEMENT_3D('',#5695,#4486,#4487) ;
#4038=AXIS2_PLACEMENT_3D('',#5696,#4488,#4489) ;
#4039=AXIS2_PLACEMENT_3D('',#5699,#4491,#4492) ;
#4040=AXIS2_PLACEMENT_3D('',#5700,#4493,#4494) ;
#4041=AXIS2_PLACEMENT_3D('',#5702,#4495,#4496) ;
#4042=AXIS2_PLACEMENT_3D('',#5705,#4498,#4499) ;
#4043=AXIS2_PLACEMENT_3D('',#5706,#4500,#4501) ;
#4044=AXIS2_PLACEMENT_3D('',#5709,#4503,#4504) ;
#4045=AXIS2_PLACEMENT_3D('',#5710,#4505,#4506) ;
#4046=AXIS2_PLACEMENT_3D('',#5718,#4510,#4511) ;
#4047=AXIS2_PLACEMENT_3D('',#5730,#4517,#4518) ;
#4048=AXIS2_PLACEMENT_3D('',#5734,#4520,#4521) ;
#4049=AXIS2_PLACEMENT_3D('',#5742,#4525,#4526) ;
#4050=AXIS2_PLACEMENT_3D('',#5746,#4528,#4529) ;
#4051=AXIS2_PLACEMENT_3D('',#5758,#4535,#4536) ;
#4052=AXIS2_PLACEMENT_3D('',#5760,#4538,#4539) ;
#4053=AXIS2_PLACEMENT_3D('',#5764,#4541,#4542) ;
#4054=AXIS2_PLACEMENT_3D('',#5766,#4544,#4545) ;
#4055=AXIS2_PLACEMENT_3D('',#5770,#4548,#4549) ;
#4056=AXIS2_PLACEMENT_3D('',#5772,#4550,#4551) ;
#4057=AXIS2_PLACEMENT_3D('',#5774,#4553,#4554) ;
#4058=AXIS2_PLACEMENT_3D('',#5778,#4557,#4558) ;
#4059=AXIS2_PLACEMENT_3D('',#5780,#4559,#4560) ;
#4060=AXIS2_PLACEMENT_3D('',#5782,#4562,#4563) ;
#4061=AXIS2_PLACEMENT_3D('',#5786,#4566,#4567) ;
#4062=AXIS2_PLACEMENT_3D('',#5788,#4568,#4569) ;
#4063=AXIS2_PLACEMENT_3D('',#5790,#4571,#4572) ;
#4064=AXIS2_PLACEMENT_3D('',#5794,#4575,#4576) ;
#4065=AXIS2_PLACEMENT_3D('',#5796,#4577,#4578) ;
#4066=AXIS2_PLACEMENT_3D('',#5798,#4580,#4581) ;
#4067=AXIS2_PLACEMENT_3D('',#5802,#4584,#4585) ;
#4068=AXIS2_PLACEMENT_3D('',#5804,#4586,#4587) ;
#4069=AXIS2_PLACEMENT_3D('',#5806,#4589,#4590) ;
#4070=AXIS2_PLACEMENT_3D('',#5810,#4593,#4594) ;
#4071=AXIS2_PLACEMENT_3D('',#5812,#4595,#4596) ;
#4072=AXIS2_PLACEMENT_3D('',#5814,#4598,#4599) ;
#4073=AXIS2_PLACEMENT_3D('',#5818,#4602,#4603) ;
#4074=AXIS2_PLACEMENT_3D('',#5820,#4604,#4605) ;
#4075=AXIS2_PLACEMENT_3D('',#5822,#4607,#4608) ;
#4076=AXIS2_PLACEMENT_3D('',#5826,#4611,#4612) ;
#4077=AXIS2_PLACEMENT_3D('',#5828,#4613,#4614) ;
#4078=AXIS2_PLACEMENT_3D('',#5830,#4616,#4617) ;
#4079=AXIS2_PLACEMENT_3D('',#5834,#4620,#4621) ;
#4080=AXIS2_PLACEMENT_3D('',#5836,#4622,#4623) ;
#4081=AXIS2_PLACEMENT_3D('',#5838,#4625,#4626) ;
#4082=AXIS2_PLACEMENT_3D('',#5842,#4629,#4630) ;
#4083=AXIS2_PLACEMENT_3D('',#5844,#4631,#4632) ;
#4084=AXIS2_PLACEMENT_3D('',#5846,#4634,#4635) ;
#4085=AXIS2_PLACEMENT_3D('',#5850,#4638,#4639) ;
#4086=AXIS2_PLACEMENT_3D('',#5852,#4640,#4641) ;
#4087=AXIS2_PLACEMENT_3D('',#5854,#4643,#4644) ;
#4088=AXIS2_PLACEMENT_3D('',#5858,#4647,#4648) ;
#4089=AXIS2_PLACEMENT_3D('',#5860,#4649,#4650) ;
#4090=AXIS2_PLACEMENT_3D('',#5862,#4652,#4653) ;
#4091=AXIS2_PLACEMENT_3D('',#5866,#4656,#4657) ;
#4092=AXIS2_PLACEMENT_3D('',#5868,#4658,#4659) ;
#4093=AXIS2_PLACEMENT_3D('',#5870,#4661,#4662) ;
#4094=AXIS2_PLACEMENT_3D('',#5874,#4665,#4666) ;
#4095=AXIS2_PLACEMENT_3D('',#5876,#4667,#4668) ;
#4096=AXIS2_PLACEMENT_3D('',#5878,#4670,#4671) ;
#4097=AXIS2_PLACEMENT_3D('',#5882,#4674,#4675) ;
#4098=AXIS2_PLACEMENT_3D('',#5884,#4676,#4677) ;
#4099=AXIS2_PLACEMENT_3D('',#5886,#4679,#4680) ;
#4100=AXIS2_PLACEMENT_3D('',#5890,#4683,#4684) ;
#4101=AXIS2_PLACEMENT_3D('',#5894,#4687,#4688) ;
#4102=AXIS2_PLACEMENT_3D('',#5899,#4690,#4691) ;
#4103=AXIS2_PLACEMENT_3D('',#5911,#4697,#4698) ;
#4104=AXIS2_PLACEMENT_3D('',#5915,#4700,#4701) ;
#4105=AXIS2_PLACEMENT_3D('',#5923,#4705,#4706) ;
#4106=AXIS2_PLACEMENT_3D('',#5927,#4708,#4709) ;
#4107=AXIS2_PLACEMENT_3D('',#5939,#4715,#4716) ;
#4108=AXIS2_PLACEMENT_3D('',#5944,#4720,#4721) ;
#4109=AXIS2_PLACEMENT_3D('',#5947,#4722,#4723) ;
#4110=AXIS2_PLACEMENT_3D('',#5950,#4726,#4727) ;
#4111=AXIS2_PLACEMENT_3D('',#5953,#4728,#4729) ;
#4112=AXIS2_PLACEMENT_3D('',#5956,#4732,#4733) ;
#4113=AXIS2_PLACEMENT_3D('',#5959,#4734,#4735) ;
#4114=AXIS2_PLACEMENT_3D('',#5962,#4738,#4739) ;
#4115=AXIS2_PLACEMENT_3D('',#5965,#4740,#4741) ;
#4116=AXIS2_PLACEMENT_3D('',#5968,#4744,#4745) ;
#4117=AXIS2_PLACEMENT_3D('',#5971,#4746,#4747) ;
#4118=AXIS2_PLACEMENT_3D('',#5974,#4750,#4751) ;
#4119=AXIS2_PLACEMENT_3D('',#5977,#4752,#4753) ;
#4120=AXIS2_PLACEMENT_3D('',#5980,#4756,#4757) ;
#4121=AXIS2_PLACEMENT_3D('',#5984,#4760,#4761) ;
#4122=AXIS2_PLACEMENT_3D('',#5986,#4763,#4764) ;
#4123=AXIS2_PLACEMENT_3D('',#5988,#4766,#4767) ;
#4124=AXIS2_PLACEMENT_3D('',#5992,#4770,#4771) ;
#4125=AXIS2_PLACEMENT_3D('',#5994,#4773,#4774) ;
#4126=AXIS2_PLACEMENT_3D('',#5996,#4776,#4777) ;
#4127=AXIS2_PLACEMENT_3D('',#6001,#4780,#4781) ;
#4128=AXIS2_PLACEMENT_3D('',#6002,#4782,#4783) ;
#4129=AXIS2_PLACEMENT_3D('',#6006,#4786,#4787) ;
#4130=AXIS2_PLACEMENT_3D('',#6009,#4789,#4790) ;
#4131=AXIS2_PLACEMENT_3D('',#6010,#4791,#4792) ;
#4132=AXIS2_PLACEMENT_3D('',#6014,#4795,#4796) ;
#4133=AXIS2_PLACEMENT_3D('',#6018,#4799,#4800) ;
#4134=AXIS2_PLACEMENT_3D('',#6019,#4801,#4802) ;
#4135=AXIS2_PLACEMENT_3D('',#6020,#4803,#4804) ;
#4136=AXIS2_PLACEMENT_3D('',#6024,#4807,#4808) ;
#4137=AXIS2_PLACEMENT_3D('',#6027,#4810,#4811) ;
#4138=AXIS2_PLACEMENT_3D('',#6028,#4812,#4813) ;
#4139=AXIS2_PLACEMENT_3D('',#6032,#4816,#4817) ;
#4140=AXIS2_PLACEMENT_3D('',#6036,#4820,#4821) ;
#4141=AXIS2_PLACEMENT_3D('',#6037,#4822,#4823) ;
#4142=AXIS2_PLACEMENT_3D('',#6038,#4824,#4825) ;
#4143=AXIS2_PLACEMENT_3D('',#6042,#4828,#4829) ;
#4144=AXIS2_PLACEMENT_3D('',#6045,#4831,#4832) ;
#4145=AXIS2_PLACEMENT_3D('',#6046,#4833,#4834) ;
#4146=AXIS2_PLACEMENT_3D('',#6050,#4837,#4838) ;
#4147=AXIS2_PLACEMENT_3D('',#6053,#4840,#4841) ;
#4148=AXIS2_PLACEMENT_3D('',#6054,#4842,#4843) ;
#4149=AXIS2_PLACEMENT_3D('',#6058,#4846,#4847) ;
#4150=AXIS2_PLACEMENT_3D('',#6061,#4849,#4850) ;
#4151=AXIS2_PLACEMENT_3D('',#6062,#4851,#4852) ;
#4152=AXIS2_PLACEMENT_3D('',#6066,#4855,#4856) ;
#4153=AXIS2_PLACEMENT_3D('',#6070,#4859,#4860) ;
#4154=AXIS2_PLACEMENT_3D('',#6071,#4861,#4862) ;
#4155=AXIS2_PLACEMENT_3D('',#6072,#4863,#4864) ;
#4156=AXIS2_PLACEMENT_3D('',#6076,#4867,#4868) ;
#4157=AXIS2_PLACEMENT_3D('',#6080,#4871,#4872) ;
#4158=AXIS2_PLACEMENT_3D('',#6081,#4873,#4874) ;
#4159=AXIS2_PLACEMENT_3D('',#6082,#4875,#4876) ;
#4160=AXIS2_PLACEMENT_3D('',#6085,#4879,#4880) ;
#4161=AXIS2_PLACEMENT_3D('',#6087,#4882,#4883) ;
#4162=AXIS2_PLACEMENT_3D('',#6089,#4885,#4886) ;
#4163=AXIS2_PLACEMENT_3D('',#6091,#4888,#4889) ;
#4164=AXIS2_PLACEMENT_3D('',#6093,#4891,#4892) ;
#4165=AXIS2_PLACEMENT_3D('',#6095,#4894,#4895) ;
#4166=AXIS2_PLACEMENT_3D('',#6097,#4897,#4898) ;
#4167=AXIS2_PLACEMENT_3D('',#6099,#4900,#4901) ;
#4168=AXIS2_PLACEMENT_3D('',#6101,#4903,#4904) ;
#4169=AXIS2_PLACEMENT_3D('',#6103,#4906,#4907) ;
#4170=AXIS2_PLACEMENT_3D('',#6105,#4909,#4910) ;
#4171=AXIS2_PLACEMENT_3D('',#6107,#4912,#4913) ;
#4172=AXIS2_PLACEMENT_3D('',#6109,#4915,#4916) ;
#4173=AXIS2_PLACEMENT_3D('',#6111,#4918,#4919) ;
#4174=AXIS2_PLACEMENT_3D('',#6113,#4921,#4922) ;
#4175=AXIS2_PLACEMENT_3D('',#6115,#4924,#4925) ;
#4176=AXIS2_PLACEMENT_3D('',#6117,#4927,#4928) ;
#4177=AXIS2_PLACEMENT_3D('',#6119,#4930,#4931) ;
#4178=AXIS2_PLACEMENT_3D('',#6121,#4933,#4934) ;
#4179=AXIS2_PLACEMENT_3D('',#6123,#4936,#4937) ;
#4180=AXIS2_PLACEMENT_3D('',#6125,#4939,#4940) ;
#4181=AXIS2_PLACEMENT_3D('',#6127,#4942,#4943) ;
#4182=AXIS2_PLACEMENT_3D('',#6129,#4945,#4946) ;
#4183=AXIS2_PLACEMENT_3D('',#6131,#4948,#4949) ;
#4184=AXIS2_PLACEMENT_3D('',#6133,#4951,#4952) ;
#4185=AXIS2_PLACEMENT_3D('',#6135,#4954,#4955) ;
#4186=AXIS2_PLACEMENT_3D('',#6137,#4957,#4958) ;
#4187=AXIS2_PLACEMENT_3D('',#6139,#4960,#4961) ;
#4188=AXIS2_PLACEMENT_3D('',#6141,#4963,#4964) ;
#4189=AXIS2_PLACEMENT_3D('',#6143,#4966,#4967) ;
#4190=AXIS2_PLACEMENT_3D('',#6145,#4969,#4970) ;
#4191=AXIS2_PLACEMENT_3D('',#6146,#4971,#4972) ;
#4439=DIRECTION('axis',(0.,0.,1.)) ;
#4440=DIRECTION('refdir',(1.,0.,0.)) ;
#4441=DIRECTION('center_axis',(0.,0.,1.)) ;
#4442=DIRECTION('ref_axis',(0.999199679743744,0.0399999999999898,0.)) ;
#4443=DIRECTION('center_axis',(0.,0.,1.)) ;
#4444=DIRECTION('ref_axis',(-1.,0.,0.)) ;
#4445=DIRECTION('',(0.,0.,1.)) ;
#4446=DIRECTION('center_axis',(0.,0.,1.)) ;
#4447=DIRECTION('ref_axis',(-1.,0.,0.)) ;
#4448=DIRECTION('',(0.,0.,1.)) ;
#4449=DIRECTION('center_axis',(-5.3290705182E-15,2.6645352591E-15,-1.)) ;
#4450=DIRECTION('ref_axis',(9.63812363252714E-14,1.,2.66453525909949E-15)) ;
#4451=DIRECTION('center_axis',(3.49912784066E-16,5.43154451424E-16,1.)) ;
#4452=DIRECTION('ref_axis',(-1.,1.113901422397E-48,3.49912784066E-16)) ;
#4453=DIRECTION('center_axis',(-5.3290705182E-15,2.6645352591E-15,1.)) ;
#4454=DIRECTION('ref_axis',(-9.67975699595058E-14,1.,-2.66453525910052E-15)) ;
#4455=DIRECTION('center_axis',(-3.49912784066E-16,-5.43154451424E-16,1.)) ;
#4456=DIRECTION('ref_axis',(-1.,1.113901422397E-48,-3.49912784066E-16)) ;
#4457=DIRECTION('center_axis',(0.,1.,0.)) ;
#4458=DIRECTION('ref_axis',(0.877582561890372,0.,-0.479425538604204)) ;
#4459=DIRECTION('center_axis',(0.,1.,0.)) ;
#4460=DIRECTION('ref_axis',(0.,0.,-1.)) ;
#4461=DIRECTION('',(0.,1.,0.)) ;
#4462=DIRECTION('center_axis',(0.,1.,0.)) ;
#4463=DIRECTION('ref_axis',(0.,0.,-1.)) ;
#4464=DIRECTION('center_axis',(-1.30266168223E-13,1.,1.71714494475E-13)) ;
#4465=DIRECTION('ref_axis',(0.877582561890372,1.96643631636608E-13,-0.479425538604204)) ;
#4466=DIRECTION('',(-0.62054458056418,0.707106781186018,0.339005049421354)) ;
#4467=DIRECTION('center_axis',(4.23048538083E-14,1.,7.74385154649E-14)) ;
#4468=DIRECTION('ref_axis',(4.65739899425144E-44,7.74385154649E-14,-1.)) ;
#4469=DIRECTION('center_axis',(0.,1.,0.)) ;
#4470=DIRECTION('ref_axis',(0.877582561890372,0.,-0.479425538604204)) ;
#4471=DIRECTION('center_axis',(0.,1.,0.)) ;
#4472=DIRECTION('ref_axis',(0.,0.,-1.)) ;
#4473=DIRECTION('',(0.,1.,0.)) ;
#4474=DIRECTION('center_axis',(0.,1.,0.)) ;
#4475=DIRECTION('ref_axis',(0.,0.,-1.)) ;
#4476=DIRECTION('center_axis',(-1.30266168223E-13,1.,1.74675089208E-13)) ;
#4477=DIRECTION('ref_axis',(0.877582561890372,1.98063016361065E-13,-0.479425538604204)) ;
#4478=DIRECTION('',(-0.62054458056418,0.707106781186017,0.339005049421356)) ;
#4479=DIRECTION('center_axis',(4.35504810908E-14,1.,7.97186209114E-14)) ;
#4480=DIRECTION('ref_axis',(2.58022100039044E-43,7.97186209114E-14,-1.)) ;
#4481=DIRECTION('center_axis',(0.,1.,0.)) ;
#4482=DIRECTION('ref_axis',(0.877582561890372,0.,-0.479425538604204)) ;
#4483=DIRECTION('center_axis',(0.,1.,0.)) ;
#4484=DIRECTION('ref_axis',(0.,0.,-1.)) ;
#4485=DIRECTION('',(0.,1.,0.)) ;
#4486=DIRECTION('center_axis',(0.,1.,0.)) ;
#4487=DIRECTION('ref_axis',(0.,0.,-1.)) ;
#4488=DIRECTION('center_axis',(-1.18423789293E-13,1.,1.7763568394E-13)) ;
#4489=DIRECTION('ref_axis',(0.877582561890372,1.89089735844777E-13,-0.479425538604204)) ;
#4490=DIRECTION('',(-0.620544580564171,0.707106781186024,0.339005049421358)) ;
#4491=DIRECTION('center_axis',(4.75180655168E-14,1.,8.6981235488E-14)) ;
#4492=DIRECTION('ref_axis',(-9.16589391413786E-44,8.6981235488E-14,-1.)) ;
#4493=DIRECTION('center_axis',(0.,1.,0.)) ;
#4494=DIRECTION('ref_axis',(0.877582561890372,0.,-0.479425538604204)) ;
#4495=DIRECTION('center_axis',(0.,1.,0.)) ;
#4496=DIRECTION('ref_axis',(0.,0.,-1.)) ;
#4497=DIRECTION('',(0.,1.,0.)) ;
#4498=DIRECTION('center_axis',(0.,1.,0.)) ;
#4499=DIRECTION('ref_axis',(0.,0.,-1.)) ;
#4500=DIRECTION('center_axis',(-1.18423789293E-13,1.,1.83556873405E-13)) ;
#4501=DIRECTION('ref_axis',(0.877582561890372,1.91928505293212E-13,-0.479425538604204)) ;
#4502=DIRECTION('',(-0.620544580564171,0.707106781186022,0.339005049421363)) ;
#4503=DIRECTION('center_axis',(5.00093200818E-14,1.,9.15414463809E-14)) ;
#4504=DIRECTION('ref_axis',(-7.43578035279155E-44,9.15414463809E-14,-1.)) ;
#4505=DIRECTION('center_axis',(0.,0.,1.)) ;
#4506=DIRECTION('ref_axis',(1.,0.,0.)) ;
#4507=DIRECTION('',(1.,0.,0.)) ;
#4508=DIRECTION('',(-1.,0.,0.)) ;
#4509=DIRECTION('',(0.,1.,0.)) ;
#4510=DIRECTION('center_axis',(-9.63097017110531E-7,6.43563312525601E-7,
-0.999999999999329)) ;
#4511=DIRECTION('ref_axis',(-0.707106621415537,0.70710694095661,1.13608036309705E-6)) ;
#4512=DIRECTION('',(0.707106781186548,0.707106781186548,0.)) ;
#4513=DIRECTION('',(0.,1.,0.)) ;
#4514=DIRECTION('',(0.707106781186548,-0.707106781186548,0.)) ;
#4515=DIRECTION('',(1.,0.,0.)) ;
#4516=DIRECTION('',(0.707106781186548,0.707106781186548,0.)) ;
#4517=DIRECTION('center_axis',(2.25942303733386E-7,-1.13593817941397E-6,
-0.999999999999329)) ;
#4518=DIRECTION('ref_axis',(-2.25947536598826E-7,-0.999999999999329,1.13593812836286E-6)) ;
#4519=DIRECTION('',(1.,0.,0.)) ;
#4520=DIRECTION('center_axis',(-6.43554037258066E-7,-9.63074619200789E-7,
-0.999999999999329)) ;
#4521=DIRECTION('ref_axis',(-0.707106940950062,-0.707106621422085,1.13605796678281E-6)) ;
#4522=DIRECTION('',(0.707106781186548,-0.707106781186548,0.)) ;
#4523=DIRECTION('',(1.,0.,0.)) ;
#4524=DIRECTION('',(-0.707106781186548,-0.707106781186548,0.)) ;
#4525=DIRECTION('center_axis',(3.96642434162338E-7,-5.93533143460979E-7,
-0.999999999999745)) ;
#4526=DIRECTION('ref_axis',(-3.24285719155748E-7,-0.999999999999771,5.93533014835517E-7)) ;
#4527=DIRECTION('',(1.,0.,0.)) ;
#4528=DIRECTION('center_axis',(-1.39239436415965E-7,-7.00115564002718E-7,
-0.999999999999745)) ;
#4529=DIRECTION('ref_axis',(-0.707107010481907,-0.707106551890865,5.9351348401252E-7)) ;
#4530=DIRECTION('',(-0.707106781186548,0.707106781186548,0.)) ;
#4531=DIRECTION('',(1.,0.,0.)) ;
#4532=DIRECTION('',(-0.707106781186548,-0.707106781186548,0.)) ;
#4533=DIRECTION('',(0.,1.,0.)) ;
#4534=DIRECTION('',(-0.707106781186548,0.707106781186548,0.)) ;
#4535=DIRECTION('center_axis',(5.93533045622587E-7,3.96642398122336E-7,
-0.999999999999745)) ;
#4536=DIRECTION('ref_axis',(0.999999999999771,-3.24285692193144E-7,5.93532916997148E-7)) ;
#4537=DIRECTION('',(0.,1.,0.)) ;
#4538=DIRECTION('center_axis',(-6.27646083255E-12,2.93098878501E-12,1.)) ;
#4539=DIRECTION('ref_axis',(-0.987688340594861,-0.156434465041978,-5.74067952188287E-12)) ;
#4540=DIRECTION('',(-0.707106781185048,1.4361112355401E-12,0.707106781188048)) ;
#4541=DIRECTION('center_axis',(6.06458601694E-13,-3.82902891499E-12,-1.)) ;
#4542=DIRECTION('ref_axis',(1.,1.11960132041635E-40,6.06458601694E-13)) ;
#4543=DIRECTION('',(-0.50000000000309,0.49999999999609,0.707106781187127)) ;
#4544=DIRECTION('center_axis',(0.49999999999984,-0.49999999999984,0.707106781186774)) ;
#4545=DIRECTION('ref_axis',(0.707106781186547,0.707106781186548,3.33066907361881E-16)) ;
#4546=DIRECTION('',(0.707106781186548,0.707106781186548,0.)) ;
#4547=DIRECTION('',(-0.49999999999984,0.49999999999984,0.707106781186774)) ;
#4548=DIRECTION('center_axis',(1.18423789293E-14,0.,-1.)) ;
#4549=DIRECTION('ref_axis',(0.98768834059517,0.156434465040027,1.16965795933795E-14)) ;
#4550=DIRECTION('center_axis',(2.89803640077E-16,-1.8297481715E-15,-1.)) ;
#4551=DIRECTION('ref_axis',(1.,2.40832247656156E-47,2.89803640077E-16)) ;
#4552=DIRECTION('',(0.707106781186548,0.,-0.707106781186548)) ;
#4553=DIRECTION('center_axis',(0.707106781186548,0.,0.707106781186548)) ;
#4554=DIRECTION('ref_axis',(0.,1.,0.)) ;
#4555=DIRECTION('',(0.,1.,0.)) ;
#4556=DIRECTION('',(-0.707106781186548,0.,0.707106781186548)) ;
#4557=DIRECTION('center_axis',(-1.18423789293E-14,-1.18423789293E-14,-1.)) ;
#4558=DIRECTION('ref_axis',(0.587785252292138,0.809016994375191,-1.65414614943321E-14)) ;
#4559=DIRECTION('center_axis',(-2.11955181157E-15,1.53994453142E-15,-1.)) ;
#4560=DIRECTION('ref_axis',(1.,-2.00835703363761E-46,-2.11955181157E-15)) ;
#4561=DIRECTION('',(0.49999999999984,0.49999999999984,-0.707106781186774)) ;
#4562=DIRECTION('center_axis',(-0.49999999999984,-0.49999999999984,-0.707106781186774)) ;
#4563=DIRECTION('ref_axis',(0.707106781186547,-0.707106781186548,3.33066907361881E-16)) ;
#4564=DIRECTION('',(0.707106781186548,-0.707106781186548,0.)) ;
#4565=DIRECTION('',(-0.49999999999984,-0.49999999999984,0.707106781186774)) ;
#4566=DIRECTION('center_axis',(0.,1.18423789293E-14,-1.)) ;
#4567=DIRECTION('ref_axis',(-0.156434465040027,0.98768834059517,1.16965795933795E-14)) ;
#4568=DIRECTION('center_axis',(1.8297481715E-15,2.89803640077E-16,-1.)) ;
#4569=DIRECTION('ref_axis',(1.,-2.40832247656156E-47,1.8297481715E-15)) ;
#4570=DIRECTION('',(0.,0.707106781186548,-0.707106781186548)) ;
#4571=DIRECTION('center_axis',(0.,-0.707106781186548,-0.707106781186548)) ;
#4572=DIRECTION('ref_axis',(1.,0.,0.)) ;
#4573=DIRECTION('',(1.,0.,0.)) ;
#4574=DIRECTION('',(0.,-0.707106781186548,0.707106781186548)) ;
#4575=DIRECTION('center_axis',(1.18423789293E-14,-1.18423789293E-14,-1.)) ;
#4576=DIRECTION('ref_axis',(-0.809016994375191,0.587785252292138,-1.65414614943321E-14)) ;
#4577=DIRECTION('center_axis',(-1.53994453142E-15,-2.11955181157E-15,-1.)) ;
#4578=DIRECTION('ref_axis',(1.,2.00835703363761E-46,-1.53994453142E-15)) ;
#4579=DIRECTION('',(-0.49999999999984,0.49999999999984,-0.707106781186774)) ;
#4580=DIRECTION('center_axis',(0.49999999999984,-0.49999999999984,-0.707106781186774)) ;
#4581=DIRECTION('ref_axis',(0.707106781186547,0.707106781186548,-3.33066907361881E-16)) ;
#4582=DIRECTION('',(0.707106781186548,0.707106781186548,0.)) ;
#4583=DIRECTION('',(0.49999999999984,-0.49999999999984,0.707106781186774)) ;
#4584=DIRECTION('center_axis',(2.37439697533E-12,-6.52515079006E-12,1.)) ;
#4585=DIRECTION('ref_axis',(0.809016994376012,-0.587785252291009,-5.75631490780926E-12)) ;
#4586=DIRECTION('center_axis',(2.28255961007E-12,3.14167377971E-12,-1.)) ;
#4587=DIRECTION('ref_axis',(1.,-2.81265537546077E-40,2.28255961007E-12)) ;
#4588=DIRECTION('',(4.97823982232033E-12,-0.707106781186048,0.707106781187048)) ;
#4589=DIRECTION('center_axis',(0.,-0.707106781186548,-0.707106781186548)) ;
#4590=DIRECTION('ref_axis',(1.,0.,0.)) ;
#4591=DIRECTION('',(1.,0.,0.)) ;
#4592=DIRECTION('',(0.,-0.707106781186548,0.707106781186548)) ;
#4593=DIRECTION('center_axis',(-2.93394937974E-12,-6.28830321148E-12,1.)) ;
#4594=DIRECTION('ref_axis',(0.156434465041978,-0.987688340594861,-5.75191296242415E-12)) ;
#4595=DIRECTION('center_axis',(3.83374680699E-12,6.07205842377E-13,-1.)) ;
#4596=DIRECTION('ref_axis',(1.,-1.49541384440967E-40,3.83374680699E-12)) ;
#4597=DIRECTION('',(-0.49999999999609,-0.50000000000309,0.707106781187127)) ;
#4598=DIRECTION('center_axis',(-0.49999999999984,-0.49999999999984,-0.707106781186774)) ;
#4599=DIRECTION('ref_axis',(0.707106781186547,-0.707106781186548,3.33066907361881E-16)) ;
#4600=DIRECTION('',(0.707106781186548,-0.707106781186548,0.)) ;
#4601=DIRECTION('',(-0.49999999999984,-0.49999999999984,0.707106781186774)) ;
#4602=DIRECTION('center_axis',(2.96059473233E-15,1.18423789293E-14,-1.)) ;
#4603=DIRECTION('ref_axis',(-0.156434465040027,0.98768834059517,1.12334405402272E-14)) ;
#4604=DIRECTION('center_axis',(4.71789199381E-15,7.47240682951E-16,-1.)) ;
#4605=DIRECTION('ref_axis',(1.,-2.48107229741873E-46,4.71789199381E-15)) ;
#4606=DIRECTION('',(-2.09345661157866E-15,0.707106781186548,-0.707106781186548)) ;
#4607=DIRECTION('center_axis',(0.,-0.707106781186548,-0.707106781186548)) ;
#4608=DIRECTION('ref_axis',(1.,0.,0.)) ;
#4609=DIRECTION('',(1.,0.,0.)) ;
#4610=DIRECTION('',(0.,-0.707106781186548,0.707106781186548)) ;
#4611=DIRECTION('center_axis',(-5.92118946467E-15,2.36847578587E-14,-1.)) ;
#4612=DIRECTION('ref_axis',(-0.809016994375191,0.587785252292138,1.87118942772875E-14)) ;
#4613=DIRECTION('center_axis',(9.21705100259E-15,1.268618236E-14,-1.)) ;
#4614=DIRECTION('ref_axis',(1.,-1.19244796912461E-45,9.21705100259E-15)) ;
#4615=DIRECTION('',(-0.49999999999984,0.49999999999984,-0.707106781186774)) ;
#4616=DIRECTION('center_axis',(-0.49999999999984,0.49999999999984,0.707106781186774)) ;
#4617=DIRECTION('ref_axis',(-0.707106781186547,-0.707106781186548,3.33066907361881E-16)) ;
#4618=DIRECTION('',(-0.707106781186548,-0.707106781186548,0.)) ;
#4619=DIRECTION('',(0.49999999999984,-0.49999999999984,0.707106781186774)) ;
#4620=DIRECTION('center_axis',(-1.48029736617E-14,3.5527136788E-14,1.)) ;
#4621=DIRECTION('ref_axis',(0.707106781186548,-0.707106781186548,3.55887623968508E-14)) ;
#4622=DIRECTION('center_axis',(-1.03620815632E-14,-1.03620815632E-14,-1.)) ;
#4623=DIRECTION('ref_axis',(1.,7.78499045260793E-45,-1.03620815632E-14)) ;
#4624=DIRECTION('',(-3.34953057852786E-14,-0.707106781186548,0.707106781186548)) ;
#4625=DIRECTION('center_axis',(0.,-0.707106781186548,-0.707106781186548)) ;
#4626=DIRECTION('ref_axis',(1.,0.,0.)) ;
#4627=DIRECTION('',(1.,0.,0.)) ;
#4628=DIRECTION('',(0.,-0.707106781186548,0.707106781186548)) ;
#4629=DIRECTION('center_axis',(5.92118946467E-15,1.18423789293E-14,1.)) ;
#4630=DIRECTION('ref_axis',(0.156434465040027,-0.98768834059517,1.07703014870732E-14)) ;
#4631=DIRECTION('center_axis',(-7.60603581612E-15,-1.20467772583E-15,-1.)) ;
#4632=DIRECTION('ref_axis',(1.,5.2570604439658E-46,-7.60603581612E-15)) ;
#4633=DIRECTION('',(-0.49999999999984,-0.49999999999984,0.707106781186774)) ;
#4634=DIRECTION('center_axis',(0.49999999999984,0.49999999999984,0.707106781186774)) ;
#4635=DIRECTION('ref_axis',(-0.707106781186547,0.707106781186548,-3.33066907361881E-16)) ;
#4636=DIRECTION('',(-0.707106781186548,0.707106781186548,0.)) ;
#4637=DIRECTION('',(-0.49999999999984,-0.49999999999984,0.707106781186774)) ;
#4638=DIRECTION('center_axis',(1.18423789293E-14,4.73695157173E-14,-1.)) ;
#4639=DIRECTION('ref_axis',(-0.156434465040027,0.98768834059517,4.49337621610105E-14)) ;
#4640=DIRECTION('center_axis',(1.88715679752E-14,2.98896273181E-15,-1.)) ;
#4641=DIRECTION('ref_axis',(1.,-3.73441846949733E-45,1.88715679752E-14)) ;
#4642=DIRECTION('',(-8.37382644630462E-15,0.707106781186548,-0.707106781186548)) ;
#4643=DIRECTION('center_axis',(0.,-0.707106781186548,-0.707106781186548)) ;
#4644=DIRECTION('ref_axis',(1.,0.,0.)) ;
#4645=DIRECTION('',(1.,0.,0.)) ;
#4646=DIRECTION('',(0.,-0.707106781186548,0.707106781186548)) ;
#4647=DIRECTION('center_axis',(-1.18423789293E-14,3.5527136788E-14,-1.)) ;
#4648=DIRECTION('ref_axis',(-0.809016994375191,0.587785252292138,3.04630128677863E-14)) ;
#4649=DIRECTION('center_axis',(1.28027161806E-14,1.76214270839E-14,-1.)) ;
#4650=DIRECTION('ref_axis',(1.,-3.57263571433164E-45,1.28027161806E-14)) ;
#4651=DIRECTION('',(-0.49999999999984,0.49999999999984,-0.707106781186774)) ;
#4652=DIRECTION('center_axis',(-0.49999999999984,0.49999999999984,0.707106781186774)) ;
#4653=DIRECTION('ref_axis',(-0.707106781186547,-0.707106781186548,3.33066907361881E-16)) ;
#4654=DIRECTION('',(-0.707106781186548,-0.707106781186548,0.)) ;
#4655=DIRECTION('',(0.49999999999984,-0.49999999999984,0.707106781186774)) ;
#4656=DIRECTION('center_axis',(-4.73695157173E-14,1.18423789293E-14,-1.)) ;
#4657=DIRECTION('ref_axis',(-0.98768834059517,-0.156434465040027,4.49337621610105E-14)) ;
#4658=DIRECTION('center_axis',(-2.98896273181E-15,1.88715679752E-14,-1.)) ;
#4659=DIRECTION('ref_axis',(1.,3.73441846949733E-45,-2.98896273181E-15)) ;
#4660=DIRECTION('',(-0.707106781186548,-8.37382644630462E-15,-0.707106781186548)) ;
#4661=DIRECTION('center_axis',(0.707106781186548,0.,-0.707106781186548)) ;
#4662=DIRECTION('ref_axis',(0.,1.,0.)) ;
#4663=DIRECTION('',(0.,1.,0.)) ;
#4664=DIRECTION('',(0.707106781186548,0.,0.707106781186548)) ;
#4665=DIRECTION('center_axis',(-1.18423789293E-14,0.,-1.)) ;
#4666=DIRECTION('ref_axis',(-0.587785252292138,-0.809016994375191,6.9607756866977E-15)) ;
#4667=DIRECTION('center_axis',(-7.75093763616E-15,5.63138582459E-15,-1.)) ;
#4668=DIRECTION('ref_axis',(1.,1.34620891396805E-45,-7.75093763616E-15)) ;
#4669=DIRECTION('',(-0.49999999999984,-0.49999999999984,-0.707106781186774)) ;
#4670=DIRECTION('center_axis',(0.49999999999984,0.49999999999984,-0.707106781186774)) ;
#4671=DIRECTION('ref_axis',(-0.707106781186547,0.707106781186548,3.33066907361881E-16)) ;
#4672=DIRECTION('',(-0.707106781186548,0.707106781186548,0.)) ;
#4673=DIRECTION('',(0.49999999999984,0.49999999999984,0.707106781186774)) ;
#4674=DIRECTION('center_axis',(-2.36847578587E-14,-1.18423789293E-14,1.)) ;
#4675=DIRECTION('ref_axis',(0.707106781186548,0.707106781186548,2.51214793389369E-14)) ;
#4676=DIRECTION('center_axis',(5.92118946467E-15,-5.92118946467E-15,-1.)) ;
#4677=DIRECTION('ref_axis',(1.,6.22799323720626E-46,5.92118946467E-15)) ;
#4678=DIRECTION('',(0.707106781186548,-3.97756756199745E-14,0.707106781186548)) ;
#4679=DIRECTION('center_axis',(0.707106781186548,0.,-0.707106781186548)) ;
#4680=DIRECTION('ref_axis',(0.,1.,0.)) ;
#4681=DIRECTION('',(0.707106781186548,0.,0.707106781186548)) ;
#4682=DIRECTION('',(0.,1.,0.)) ;
#4683=DIRECTION('center_axis',(0.707106781186548,0.,0.707106781186548)) ;
#4684=DIRECTION('ref_axis',(0.,1.,0.)) ;
#4685=DIRECTION('',(0.,1.,0.)) ;
#4686=DIRECTION('',(-0.707106781186548,0.,0.707106781186548)) ;
#4687=DIRECTION('center_axis',(0.,0.,1.)) ;
#4688=DIRECTION('ref_axis',(1.,0.,0.)) ;
#4689=DIRECTION('',(0.,1.,0.)) ;
#4690=DIRECTION('center_axis',(-5.9353304562263E-7,-3.96642398122351E-7,
-0.999999999999745)) ;
#4691=DIRECTION('ref_axis',(0.999999999999771,-3.24285666816574E-7,-5.93532916997201E-7)) ;
#4692=DIRECTION('',(-0.707106781186548,0.707106781186548,0.)) ;
#4693=DIRECTION('',(0.,1.,0.)) ;
#4694=DIRECTION('',(-0.707106781186548,-0.707106781186548,0.)) ;
#4695=DIRECTION('',(1.,0.,0.)) ;
#4696=DIRECTION('',(-0.707106781186548,0.707106781186548,0.)) ;
#4697=DIRECTION('center_axis',(1.39239491916582E-7,7.00115676332798E-7,
-0.999999999999745)) ;
#4698=DIRECTION('ref_axis',(-0.707107010481932,-0.707106551890839,-5.93513602686716E-7)) ;
#4699=DIRECTION('',(1.,0.,0.)) ;
#4700=DIRECTION('center_axis',(-3.96642440063609E-7,5.93533152292858E-7,
-0.999999999999745)) ;
#4701=DIRECTION('ref_axis',(-3.24285714397637E-7,-0.999999999999771,-5.93533023667397E-7)) ;
#4702=DIRECTION('',(-0.707106781186548,-0.707106781186548,0.)) ;
#4703=DIRECTION('',(1.,0.,0.)) ;
#4704=DIRECTION('',(0.707106781186548,-0.707106781186548,0.)) ;
#4705=DIRECTION('center_axis',(6.4354811537276E-7,9.63053640304665E-7,-0.999999999999329)) ;
#4706=DIRECTION('ref_axis',(-0.707106940957591,-0.707106621414556,-1.13603894505784E-6)) ;
#4707=DIRECTION('',(1.,0.,0.)) ;
#4708=DIRECTION('center_axis',(-2.25931656503166E-7,1.13591913526646E-6,
-0.999999999999329)) ;
#4709=DIRECTION('ref_axis',(-2.25958188412347E-7,-0.999999999999329,-1.13591908421535E-6)) ;
#4710=DIRECTION('',(0.707106781186548,0.707106781186548,0.)) ;
#4711=DIRECTION('',(1.,0.,0.)) ;
#4712=DIRECTION('',(0.707106781186548,-0.707106781186548,0.)) ;
#4713=DIRECTION('',(0.,1.,0.)) ;
#4714=DIRECTION('',(0.707106781186548,0.707106781186548,0.)) ;
#4715=DIRECTION('center_axis',(9.63097017110531E-7,-6.43563312525601E-7,
-0.999999999999329)) ;
#4716=DIRECTION('ref_axis',(-0.707106621415537,0.70710694095661,-1.13608036309705E-6)) ;
#4717=DIRECTION('',(0.,1.,0.)) ;
#4718=DIRECTION('',(-1.,0.,0.)) ;
#4719=DIRECTION('',(1.,0.,0.)) ;
#4720=DIRECTION('center_axis',(0.,0.,1.)) ;
#4721=DIRECTION('ref_axis',(0.,-1.,0.)) ;
#4722=DIRECTION('center_axis',(0.,0.,1.)) ;
#4723=DIRECTION('ref_axis',(-1.,0.,0.)) ;
#4724=DIRECTION('',(0.,0.,1.)) ;
#4725=DIRECTION('',(0.,0.,1.)) ;
#4726=DIRECTION('center_axis',(0.,0.,1.)) ;
#4727=DIRECTION('ref_axis',(-0.707106781186548,-0.707106781186548,0.)) ;
#4728=DIRECTION('center_axis',(0.,0.,1.)) ;
#4729=DIRECTION('ref_axis',(-1.,0.,0.)) ;
#4730=DIRECTION('',(0.,0.,1.)) ;
#4731=DIRECTION('',(0.,0.,1.)) ;
#4732=DIRECTION('center_axis',(0.,0.,1.)) ;
#4733=DIRECTION('ref_axis',(0.,-1.,0.)) ;
#4734=DIRECTION('center_axis',(0.,0.,1.)) ;
#4735=DIRECTION('ref_axis',(-1.,0.,0.)) ;
#4736=DIRECTION('',(0.,0.,1.)) ;
#4737=DIRECTION('',(0.,0.,1.)) ;
#4738=DIRECTION('center_axis',(0.,0.,1.)) ;
#4739=DIRECTION('ref_axis',(-0.707106781186548,-0.707106781186548,0.)) ;
#4740=DIRECTION('center_axis',(0.,0.,1.)) ;
#4741=DIRECTION('ref_axis',(-1.,0.,0.)) ;
#4742=DIRECTION('',(0.,0.,1.)) ;
#4743=DIRECTION('',(0.,0.,1.)) ;
#4744=DIRECTION('center_axis',(0.,0.,1.)) ;
#4745=DIRECTION('ref_axis',(1.,0.,0.)) ;
#4746=DIRECTION('center_axis',(0.,0.,1.)) ;
#4747=DIRECTION('ref_axis',(-1.,0.,0.)) ;
#4748=DIRECTION('',(0.,0.,1.)) ;
#4749=DIRECTION('',(0.,0.,1.)) ;
#4750=DIRECTION('center_axis',(0.,0.,1.)) ;
#4751=DIRECTION('ref_axis',(-0.707106781186548,0.707106781186548,0.)) ;
#4752=DIRECTION('center_axis',(0.,0.,1.)) ;
#4753=DIRECTION('ref_axis',(-1.,0.,0.)) ;
#4754=DIRECTION('',(0.,0.,1.)) ;
#4755=DIRECTION('',(0.,0.,1.)) ;
#4756=DIRECTION('center_axis',(-1.,0.,0.)) ;
#4757=DIRECTION('ref_axis',(0.,-1.,0.)) ;
#4758=DIRECTION('',(0.,1.,0.)) ;
#4759=DIRECTION('',(0.,0.,1.)) ;
#4760=DIRECTION('center_axis',(0.,1.,0.)) ;
#4761=DIRECTION('ref_axis',(-1.,0.,0.)) ;
#4762=DIRECTION('',(1.,0.,0.)) ;
#4763=DIRECTION('center_axis',(0.,1.,0.)) ;
#4764=DIRECTION('ref_axis',(-1.,0.,0.)) ;
#4765=DIRECTION('',(1.,0.,0.)) ;
#4766=DIRECTION('center_axis',(-1.,0.,0.)) ;
#4767=DIRECTION('ref_axis',(0.,-1.,0.)) ;
#4768=DIRECTION('',(0.,0.,1.)) ;
#4769=DIRECTION('',(0.,1.,0.)) ;
#4770=DIRECTION('center_axis',(0.,-1.,0.)) ;
#4771=DIRECTION('ref_axis',(1.,0.,0.)) ;
#4772=DIRECTION('',(-0.707106781186548,0.,-0.707106781186548)) ;
#4773=DIRECTION('center_axis',(0.,-1.,0.)) ;
#4774=DIRECTION('ref_axis',(1.,0.,0.)) ;
#4775=DIRECTION('',(0.707106781186548,0.,-0.707106781186548)) ;
#4776=DIRECTION('center_axis',(0.,0.,1.)) ;
#4777=DIRECTION('ref_axis',(1.,-2.22044604925E-16,0.)) ;
#4778=DIRECTION('',(0.,0.,1.)) ;
#4779=DIRECTION('',(0.,0.,1.)) ;
#4780=DIRECTION('center_axis',(0.,0.,1.)) ;
#4781=DIRECTION('ref_axis',(-1.,0.,0.)) ;
#4782=DIRECTION('center_axis',(0.707106781186548,0.707106781186548,0.)) ;
#4783=DIRECTION('ref_axis',(-0.707106781186548,0.707106781186548,0.)) ;
#4784=DIRECTION('',(0.,0.,1.)) ;
#4785=DIRECTION('',(0.707106781186548,-0.707106781186548,0.)) ;
#4786=DIRECTION('center_axis',(0.,0.,1.)) ;
#4787=DIRECTION('ref_axis',(0.707106781186547,0.707106781186547,0.)) ;
#4788=DIRECTION('',(0.,0.,1.)) ;
#4789=DIRECTION('center_axis',(0.,0.,1.)) ;
#4790=DIRECTION('ref_axis',(-1.,0.,0.)) ;
#4791=DIRECTION('center_axis',(-0.707106781186548,0.707106781186548,0.)) ;
#4792=DIRECTION('ref_axis',(-0.707106781186548,-0.707106781186548,0.)) ;
#4793=DIRECTION('',(0.,0.,1.)) ;
#4794=DIRECTION('',(0.707106781186548,0.707106781186548,0.)) ;
#4795=DIRECTION('center_axis',(0.,1.,0.)) ;
#4796=DIRECTION('ref_axis',(-1.,0.,0.)) ;
#4797=DIRECTION('',(0.,0.,1.)) ;
#4798=DIRECTION('',(1.,0.,0.)) ;
#4799=DIRECTION('center_axis',(0.,0.,1.)) ;
#4800=DIRECTION('ref_axis',(2.22044604925E-16,1.,0.)) ;
#4801=DIRECTION('center_axis',(0.,0.,1.)) ;
#4802=DIRECTION('ref_axis',(-1.,0.,0.)) ;
#4803=DIRECTION('center_axis',(0.707106781186548,0.707106781186548,0.)) ;
#4804=DIRECTION('ref_axis',(-0.707106781186548,0.707106781186548,0.)) ;
#4805=DIRECTION('',(0.,0.,1.)) ;
#4806=DIRECTION('',(0.707106781186548,-0.707106781186548,0.)) ;
#4807=DIRECTION('center_axis',(0.,0.,1.)) ;
#4808=DIRECTION('ref_axis',(0.707106781186547,0.707106781186547,0.)) ;
#4809=DIRECTION('',(0.,0.,1.)) ;
#4810=DIRECTION('center_axis',(0.,0.,1.)) ;
#4811=DIRECTION('ref_axis',(-1.,0.,0.)) ;
#4812=DIRECTION('center_axis',(0.707106781186548,-0.707106781186548,0.)) ;
#4813=DIRECTION('ref_axis',(0.707106781186548,0.707106781186548,0.)) ;
#4814=DIRECTION('',(-0.707106781186548,-0.707106781186548,0.)) ;
#4815=DIRECTION('',(0.,0.,1.)) ;
#4816=DIRECTION('center_axis',(0.,1.,0.)) ;
#4817=DIRECTION('ref_axis',(-1.,0.,0.)) ;
#4818=DIRECTION('',(0.,0.,1.)) ;
#4819=DIRECTION('',(1.,0.,0.)) ;
#4820=DIRECTION('center_axis',(0.,0.,1.)) ;
#4821=DIRECTION('ref_axis',(-2.22044604925E-16,1.,0.)) ;
#4822=DIRECTION('center_axis',(0.,0.,1.)) ;
#4823=DIRECTION('ref_axis',(-1.,0.,0.)) ;
#4824=DIRECTION('center_axis',(-0.707106781186548,-0.707106781186548,0.)) ;
#4825=DIRECTION('ref_axis',(0.707106781186548,-0.707106781186548,0.)) ;
#4826=DIRECTION('',(-0.707106781186548,0.707106781186548,0.)) ;
#4827=DIRECTION('',(0.,0.,1.)) ;
#4828=DIRECTION('center_axis',(0.,0.,1.)) ;
#4829=DIRECTION('ref_axis',(0.707106781186547,0.707106781186547,0.)) ;
#4830=DIRECTION('',(0.,0.,1.)) ;
#4831=DIRECTION('center_axis',(0.,0.,1.)) ;
#4832=DIRECTION('ref_axis',(-1.,0.,0.)) ;
#4833=DIRECTION('center_axis',(0.,1.,0.)) ;
#4834=DIRECTION('ref_axis',(-1.,0.,0.)) ;
#4835=DIRECTION('',(0.,0.,1.)) ;
#4836=DIRECTION('',(1.,0.,0.)) ;
#4837=DIRECTION('center_axis',(0.,0.,1.)) ;
#4838=DIRECTION('ref_axis',(-1.14352971536E-14,1.,0.)) ;
#4839=DIRECTION('',(0.,0.,1.)) ;
#4840=DIRECTION('center_axis',(0.,0.,1.)) ;
#4841=DIRECTION('ref_axis',(-1.,0.,0.)) ;
#4842=DIRECTION('center_axis',(0.707106781186548,-0.707106781186548,0.)) ;
#4843=DIRECTION('ref_axis',(0.707106781186548,0.707106781186548,0.)) ;
#4844=DIRECTION('',(-0.707106781186548,-0.707106781186548,0.)) ;
#4845=DIRECTION('',(0.,0.,1.)) ;
#4846=DIRECTION('center_axis',(0.,0.,1.)) ;
#4847=DIRECTION('ref_axis',(-0.707106781186547,0.707106781186547,0.)) ;
#4848=DIRECTION('',(0.,0.,1.)) ;
#4849=DIRECTION('center_axis',(0.,0.,1.)) ;
#4850=DIRECTION('ref_axis',(-1.,0.,0.)) ;
#4851=DIRECTION('center_axis',(-0.707106781186548,0.707106781186548,0.)) ;
#4852=DIRECTION('ref_axis',(-0.707106781186548,-0.707106781186548,0.)) ;
#4853=DIRECTION('',(0.707106781186548,0.707106781186548,0.)) ;
#4854=DIRECTION('',(0.,0.,1.)) ;
#4855=DIRECTION('center_axis',(-1.,0.,0.)) ;
#4856=DIRECTION('ref_axis',(0.,-1.,0.)) ;
#4857=DIRECTION('',(0.,1.,0.)) ;
#4858=DIRECTION('',(0.,0.,1.)) ;
#4859=DIRECTION('center_axis',(0.,0.,1.)) ;
#4860=DIRECTION('ref_axis',(0.707106781186547,-0.707106781186547,0.)) ;
#4861=DIRECTION('center_axis',(0.,0.,1.)) ;
#4862=DIRECTION('ref_axis',(-1.,0.,0.)) ;
#4863=DIRECTION('center_axis',(-0.707106781186548,-0.707106781186548,0.)) ;
#4864=DIRECTION('ref_axis',(0.707106781186548,-0.707106781186548,0.)) ;
#4865=DIRECTION('',(0.,0.,1.)) ;
#4866=DIRECTION('',(-0.707106781186548,0.707106781186548,0.)) ;
#4867=DIRECTION('center_axis',(-1.,0.,0.)) ;
#4868=DIRECTION('ref_axis',(0.,-1.,0.)) ;
#4869=DIRECTION('',(0.,0.,1.)) ;
#4870=DIRECTION('',(0.,1.,0.)) ;
#4871=DIRECTION('center_axis',(0.,0.,1.)) ;
#4872=DIRECTION('ref_axis',(-1.,2.22044604925E-16,0.)) ;
#4873=DIRECTION('center_axis',(0.,0.,1.)) ;
#4874=DIRECTION('ref_axis',(-1.,0.,0.)) ;
#4875=DIRECTION('center_axis',(-6.27646083255E-12,2.93098878501E-12,-1.)) ;
#4876=DIRECTION('ref_axis',(-0.987688340594861,-0.156434465041978,5.74067952188287E-12)) ;
#4877=DIRECTION('',(-0.707106781185044,-1.06686070120007E-7,-0.707106781188043)) ;
#4878=DIRECTION('',(-0.50000000000284,0.49999999999684,-0.707106781186774)) ;
#4879=DIRECTION('center_axis',(-0.49999999999984,0.49999999999984,0.707106781186774)) ;
#4880=DIRECTION('ref_axis',(0.707106781186547,0.707106781186548,-3.33066907361881E-16)) ;
#4881=DIRECTION('',(-0.49999999999984,0.49999999999984,-0.707106781186774)) ;
#4882=DIRECTION('center_axis',(1.18423789293E-14,0.,1.)) ;
#4883=DIRECTION('ref_axis',(0.98768834059517,0.156434465040027,-1.16965795933795E-14)) ;
#4884=DIRECTION('',(0.707106781186548,0.,0.707106781186548)) ;
#4885=DIRECTION('center_axis',(-0.707106781186548,0.,0.707106781186548)) ;
#4886=DIRECTION('ref_axis',(0.,1.,0.)) ;
#4887=DIRECTION('',(-0.707106781186548,0.,-0.707106781186548)) ;
#4888=DIRECTION('center_axis',(-1.18423789293E-14,-1.18423789293E-14,1.)) ;
#4889=DIRECTION('ref_axis',(0.587785252292138,0.809016994375191,1.65414614943321E-14)) ;
#4890=DIRECTION('',(0.49999999999984,0.49999999999984,0.707106781186774)) ;
#4891=DIRECTION('center_axis',(0.49999999999984,0.49999999999984,-0.707106781186774)) ;
#4892=DIRECTION('ref_axis',(0.707106781186547,-0.707106781186548,-3.33066907361881E-16)) ;
#4893=DIRECTION('',(-0.49999999999984,-0.49999999999984,-0.707106781186774)) ;
#4894=DIRECTION('center_axis',(0.,1.18423789293E-14,1.)) ;
#4895=DIRECTION('ref_axis',(-0.156434465040027,0.98768834059517,-1.16965795933795E-14)) ;
#4896=DIRECTION('',(0.,0.707106781186548,0.707106781186548)) ;
#4897=DIRECTION('center_axis',(0.,0.707106781186548,-0.707106781186548)) ;
#4898=DIRECTION('ref_axis',(1.,0.,0.)) ;
#4899=DIRECTION('',(0.,-0.707106781186548,-0.707106781186548)) ;
#4900=DIRECTION('center_axis',(1.18423789293E-14,-1.18423789293E-14,1.)) ;
#4901=DIRECTION('ref_axis',(-0.809016994375191,0.587785252292138,1.65414614943321E-14)) ;
#4902=DIRECTION('',(-0.49999999999984,0.49999999999984,0.707106781186774)) ;
#4903=DIRECTION('center_axis',(-0.49999999999984,0.49999999999984,-0.707106781186774)) ;
#4904=DIRECTION('ref_axis',(0.707106781186547,0.707106781186548,3.33066907361881E-16)) ;
#4905=DIRECTION('',(0.49999999999984,-0.49999999999984,-0.707106781186774)) ;
#4906=DIRECTION('center_axis',(1.30266168223E-11,-2.55795384874E-11,-1.)) ;
#4907=DIRECTION('ref_axis',(0.809016994378129,-0.587785252288094,2.55740298717221E-11)) ;
#4908=DIRECTION('',(1.98962116363013E-11,-0.707106781181048,-0.707106781192048)) ;
#4909=DIRECTION('center_axis',(0.,0.707106781186548,-0.707106781186548)) ;
#4910=DIRECTION('ref_axis',(1.,0.,0.)) ;
#4911=DIRECTION('',(0.,-0.707106781186548,-0.707106781186548)) ;
#4912=DIRECTION('center_axis',(-8.86698122334E-12,-2.72966834321E-11,-1.)) ;
#4913=DIRECTION('ref_axis',(0.156434465046035,-0.987688340594219,2.55735144985301E-11)) ;
#4914=DIRECTION('',(-0.499999999982072,-0.500000000010072,-0.707106781192102)) ;
#4915=DIRECTION('center_axis',(0.49999999999984,0.49999999999984,-0.707106781186774)) ;
#4916=DIRECTION('ref_axis',(0.707106781186547,-0.707106781186548,-3.33066907361881E-16)) ;
#4917=DIRECTION('',(-0.49999999999984,-0.49999999999984,-0.707106781186774)) ;
#4918=DIRECTION('center_axis',(2.96059473233E-15,1.18423789293E-14,1.)) ;
#4919=DIRECTION('ref_axis',(-0.156434465040027,0.98768834059517,-1.12334405402272E-14)) ;
#4920=DIRECTION('',(-2.09345661157866E-15,0.707106781186548,0.707106781186548)) ;
#4921=DIRECTION('center_axis',(0.,0.707106781186548,-0.707106781186548)) ;
#4922=DIRECTION('ref_axis',(1.,0.,0.)) ;
#4923=DIRECTION('',(0.,-0.707106781186548,-0.707106781186548)) ;
#4924=DIRECTION('center_axis',(-5.92118946467E-15,2.36847578587E-14,1.)) ;
#4925=DIRECTION('ref_axis',(-0.809016994375191,0.587785252292138,-1.87118942772875E-14)) ;
#4926=DIRECTION('',(-0.49999999999984,0.49999999999984,0.707106781186774)) ;
#4927=DIRECTION('center_axis',(0.49999999999984,-0.49999999999984,0.707106781186774)) ;
#4928=DIRECTION('ref_axis',(-0.707106781186547,-0.707106781186548,-3.33066907361881E-16)) ;
#4929=DIRECTION('',(0.49999999999984,-0.49999999999984,-0.707106781186774)) ;
#4930=DIRECTION('center_axis',(-1.18423789293E-14,2.36847578587E-14,-1.)) ;
#4931=DIRECTION('ref_axis',(0.809016994375191,-0.587785252292138,-2.35022371810886E-14)) ;
#4932=DIRECTION('',(5.11457513742672E-8,-0.707106781186547,-0.707106781186547)) ;
#4933=DIRECTION('center_axis',(0.,0.707106781186548,-0.707106781186548)) ;
#4934=DIRECTION('ref_axis',(1.,0.,0.)) ;
#4935=DIRECTION('',(0.,-0.707106781186548,-0.707106781186548)) ;
#4936=DIRECTION('center_axis',(1.7763568394E-14,2.36847578587E-14,-1.)) ;
#4937=DIRECTION('ref_axis',(0.156434465040027,-0.98768834059517,-2.06143248679405E-14)) ;
#4938=DIRECTION('',(-0.499999963833839,-0.500000036165839,-0.707106781186773)) ;
#4939=DIRECTION('center_axis',(-0.49999999999984,-0.49999999999984,0.707106781186774)) ;
#4940=DIRECTION('ref_axis',(-0.707106781186547,0.707106781186548,3.33066907361881E-16)) ;
#4941=DIRECTION('',(-0.49999999999984,-0.49999999999984,-0.707106781186774)) ;
#4942=DIRECTION('center_axis',(-1.18423789293E-14,-1.18423789293E-14,1.)) ;
#4943=DIRECTION('ref_axis',(-0.156434465040027,0.98768834059517,9.84402338077319E-15)) ;
#4944=DIRECTION('',(-4.18691322315732E-15,0.707106781186548,0.707106781186548)) ;
#4945=DIRECTION('center_axis',(0.,0.707106781186548,-0.707106781186548)) ;
#4946=DIRECTION('ref_axis',(1.,0.,0.)) ;
#4947=DIRECTION('',(0.,-0.707106781186548,-0.707106781186548)) ;
#4948=DIRECTION('center_axis',(-1.18423789293E-14,3.5527136788E-14,1.)) ;
#4949=DIRECTION('ref_axis',(-0.809016994375191,0.587785252292138,-3.04630128677863E-14)) ;
#4950=DIRECTION('',(-0.49999999999984,0.49999999999984,0.707106781186774)) ;
#4951=DIRECTION('center_axis',(0.49999999999984,-0.49999999999984,0.707106781186774)) ;
#4952=DIRECTION('ref_axis',(-0.707106781186547,-0.707106781186548,-3.33066907361881E-16)) ;
#4953=DIRECTION('',(0.49999999999984,-0.49999999999984,-0.707106781186774)) ;
#4954=DIRECTION('center_axis',(1.18423789293E-14,-5.92118946467E-15,1.)) ;
#4955=DIRECTION('ref_axis',(-0.98768834059517,-0.156434465040027,1.07703014870732E-14)) ;
#4956=DIRECTION('',(-0.707106781186548,-4.18691322315732E-15,0.707106781186548)) ;
#4957=DIRECTION('center_axis',(-0.707106781186548,0.,-0.707106781186548)) ;
#4958=DIRECTION('ref_axis',(0.,1.,0.)) ;
#4959=DIRECTION('',(0.707106781186548,0.,-0.707106781186548)) ;
#4960=DIRECTION('center_axis',(-1.18423789293E-14,0.,1.)) ;
#4961=DIRECTION('ref_axis',(-0.587785252292138,-0.809016994375191,-6.9607756866977E-15)) ;
#4962=DIRECTION('',(-0.49999999999984,-0.49999999999984,0.707106781186774)) ;
#4963=DIRECTION('center_axis',(-0.49999999999984,-0.49999999999984,-0.707106781186774)) ;
#4964=DIRECTION('ref_axis',(-0.707106781186547,0.707106781186548,-3.33066907361881E-16)) ;
#4965=DIRECTION('',(0.49999999999984,0.49999999999984,-0.707106781186774)) ;
#4966=DIRECTION('center_axis',(-1.18423789293E-14,-8.881784197E-15,-1.)) ;
#4967=DIRECTION('ref_axis',(0.587785252292138,0.809016994375191,-1.41462900424437E-14)) ;
#4968=DIRECTION('',(0.707106781186547,5.11457513742672E-8,-0.707106781186547)) ;
#4969=DIRECTION('center_axis',(-0.707106781186548,0.,-0.707106781186548)) ;
#4970=DIRECTION('ref_axis',(0.,1.,0.)) ;
#4971=DIRECTION('center_axis',(-0.707106781186548,0.,0.707106781186548)) ;
#4972=DIRECTION('ref_axis',(0.,1.,0.)) ;
#5640=CARTESIAN_POINT('',(0.,0.,0.)) ;
#5641=CARTESIAN_POINT('Origin',(0.,0.,0.)) ;
#5642=CARTESIAN_POINT('',(-27.477991193,1.1,-19.)) ;
#5643=CARTESIAN_POINT('',(27.477991193,1.1,-19.)) ;
#5644=CARTESIAN_POINT('Origin',(0.,0.,-19.)) ;
#5645=CARTESIAN_POINT('',(27.477991193,1.1,19.)) ;
#5646=CARTESIAN_POINT('',(27.477991193,1.1,0.)) ;
#5647=CARTESIAN_POINT('',(-27.477991193,1.1,19.)) ;
#5648=CARTESIAN_POINT('Origin',(0.,0.,19.)) ;
#5649=CARTESIAN_POINT('',(-27.477991193,1.1,0.)) ;
#5650=CARTESIAN_POINT('Origin',(1.46549439250795E-13,-7.50510764646976E-14,
7.4999999999991)) ;
#5651=CARTESIAN_POINT('',(28.4787640181,1.1,-20.)) ;
#5652=CARTESIAN_POINT('Ctrl Pts',(27.477991192964,1.1,-19.0000000000358)) ;
#5653=CARTESIAN_POINT('Ctrl Pts',(27.969442133948,1.1,-19.4910576228772)) ;
#5654=CARTESIAN_POINT('Ctrl Pts',(28.4787640182424,1.1,-20.0000000001439)) ;
#5655=CARTESIAN_POINT('',(-28.4787640181,1.1,-20.)) ;
#5656=CARTESIAN_POINT('Ctrl Pts',(-27.4779911929642,1.1,-19.0000000000358)) ;
#5657=CARTESIAN_POINT('Ctrl Pts',(-27.9694421338791,1.1,-19.4910576228081)) ;
#5658=CARTESIAN_POINT('Ctrl Pts',(-28.4787640180994,1.1,-20.0000000000006)) ;
#5659=CARTESIAN_POINT('Origin',(8.5828066488E-28,-1.7763568394E-15,-20.)) ;
#5660=CARTESIAN_POINT('Origin',(1.46549439250795E-13,-7.50510764646976E-14,
-7.4999999999991)) ;
#5661=CARTESIAN_POINT('',(-28.4787640181,1.1,20.)) ;
#5662=CARTESIAN_POINT('',(28.4787640181,1.1,20.)) ;
#5663=CARTESIAN_POINT('Origin',(8.5828066488E-28,-1.7763568394E-15,20.)) ;
#5664=CARTESIAN_POINT('Ctrl Pts',(-27.4779911929643,1.10000000000001,19.0000000000358)) ;
#5665=CARTESIAN_POINT('Ctrl Pts',(-27.9694421339483,1.1,19.4910576228773)) ;
#5666=CARTESIAN_POINT('Ctrl Pts',(-28.4787640182428,1.1,20.0000000001439)) ;
#5667=CARTESIAN_POINT('Ctrl Pts',(27.4779911929641,1.1,19.0000000000359)) ;
#5668=CARTESIAN_POINT('Ctrl Pts',(27.969442133879,1.1,19.4910576228083)) ;
#5669=CARTESIAN_POINT('Ctrl Pts',(28.4787640180992,1.1,20.0000000000008)) ;
#5670=CARTESIAN_POINT('Origin',(35.,1.2,10.)) ;
#5671=CARTESIAN_POINT('',(32.1478566739,1.1,11.5581330005)) ;
#5672=CARTESIAN_POINT('Origin',(35.,1.1,10.)) ;
#5673=CARTESIAN_POINT('',(32.1478566739,33.1,11.5581330005)) ;
#5674=CARTESIAN_POINT('',(32.1478566738563,1.2,11.5581330004637)) ;
#5675=CARTESIAN_POINT('Origin',(35.,33.1,10.)) ;
#5676=CARTESIAN_POINT('Origin',(34.9999999999999,30.8499999999989,10.0000000000002)) ;
#5677=CARTESIAN_POINT('',(31.6213071102,33.7,11.845788275)) ;
#5678=CARTESIAN_POINT('',(34.1224174381095,30.8499999999987,10.4794255386044)) ;
#5679=CARTESIAN_POINT('Origin',(35.,33.7,10.)) ;
#5680=CARTESIAN_POINT('Origin',(35.,1.2,-10.)) ;
#5681=CARTESIAN_POINT('',(32.1478566739,1.1,-8.44186699954)) ;
#5682=CARTESIAN_POINT('Origin',(35.,1.1,-10.)) ;
#5683=CARTESIAN_POINT('',(32.1478566739,33.1,-8.44186699954)) ;
#5684=CARTESIAN_POINT('',(32.1478566738563,1.2,-8.44186699953634)) ;
#5685=CARTESIAN_POINT('Origin',(35.,33.1,-10.)) ;
#5686=CARTESIAN_POINT('Origin',(34.9999999999999,30.8499999999989,-9.99999999999983)) ;
#5687=CARTESIAN_POINT('',(31.6213071102,33.7,-8.15421172498)) ;
#5688=CARTESIAN_POINT('',(34.1224174381095,30.8499999999987,-9.52057446139563)) ;
#5689=CARTESIAN_POINT('Origin',(35.,33.7,-10.)) ;
#5690=CARTESIAN_POINT('Origin',(-35.,1.2,10.)) ;
#5691=CARTESIAN_POINT('',(-37.8521433261,1.1,11.5581330005)) ;
#5692=CARTESIAN_POINT('Origin',(-35.,1.1,10.)) ;
#5693=CARTESIAN_POINT('',(-37.8521433261,33.1,11.5581330005)) ;
#5694=CARTESIAN_POINT('',(-37.8521433261437,1.2,11.5581330004637)) ;
#5695=CARTESIAN_POINT('Origin',(-35.,33.1,10.)) ;
#5696=CARTESIAN_POINT('Origin',(-35.0000000000001,30.8499999999989,10.0000000000002)) ;
#5697=CARTESIAN_POINT('',(-38.3786928898,33.7,11.845788275)) ;
#5698=CARTESIAN_POINT('',(-35.8775825618905,30.8499999999987,10.4794255386044)) ;
#5699=CARTESIAN_POINT('Origin',(-35.,33.7,10.)) ;
#5700=CARTESIAN_POINT('Origin',(-35.,1.2,-10.)) ;
#5701=CARTESIAN_POINT('',(-37.8521433261,1.1,-8.44186699954)) ;
#5702=CARTESIAN_POINT('Origin',(-35.,1.1,-10.)) ;
#5703=CARTESIAN_POINT('',(-37.8521433261,33.1,-8.44186699954)) ;
#5704=CARTESIAN_POINT('',(-37.8521433261437,1.2,-8.44186699953634)) ;
#5705=CARTESIAN_POINT('Origin',(-35.,33.1,-10.)) ;
#5706=CARTESIAN_POINT('Origin',(-35.0000000000001,30.8499999999989,-9.99999999999982)) ;
#5707=CARTESIAN_POINT('',(-38.3786928898,33.7,-8.15421172498)) ;
#5708=CARTESIAN_POINT('',(-35.8775825618905,30.8499999999987,-9.52057446139562)) ;
#5709=CARTESIAN_POINT('Origin',(-35.,33.7,-10.)) ;
#5710=CARTESIAN_POINT('Origin',(0.,0.,20.)) ;
#5711=CARTESIAN_POINT('',(-41.85,1.1,20.)) ;
#5712=CARTESIAN_POINT('',(-35.1643820091,1.1,20.)) ;
#5713=CARTESIAN_POINT('',(41.85,1.1,20.)) ;
#5714=CARTESIAN_POINT('',(35.1643820091,1.1,20.)) ;
#5715=CARTESIAN_POINT('',(41.8500001209205,13.3686291499579,19.9999998790792)) ;
#5716=CARTESIAN_POINT('',(41.85,7.23431457505,20.)) ;
#5717=CARTESIAN_POINT('',(42.2600505063,14.3585786438,20.)) ;
#5718=CARTESIAN_POINT('Origin',(43.2499986516453,13.3686300510977,19.9999984095153)) ;
#5719=CARTESIAN_POINT('',(44.4,16.4985281374,20.)) ;
#5720=CARTESIAN_POINT('',(43.3300252532,15.4285533906,20.)) ;
#5721=CARTESIAN_POINT('',(44.4,31.4514718626,20.)) ;
#5722=CARTESIAN_POINT('',(44.4,23.975,20.)) ;
#5723=CARTESIAN_POINT('',(42.7514718626,33.1,20.)) ;
#5724=CARTESIAN_POINT('',(43.5757359313,32.2757359313,20.)) ;
#5725=CARTESIAN_POINT('',(25.2485281374,33.1,20.)) ;
#5726=CARTESIAN_POINT('',(34.,33.1,20.)) ;
#5727=CARTESIAN_POINT('',(23.6585785583632,31.5100505919387,19.9999998790932)) ;
#5728=CARTESIAN_POINT('',(24.4535533906,32.3050252532,20.)) ;
#5729=CARTESIAN_POINT('',(22.6686291501,31.1,20.)) ;
#5730=CARTESIAN_POINT('Origin',(22.6686294664262,32.4999984096667,19.9999984096869)) ;
#5731=CARTESIAN_POINT('',(11.0713708500427,31.1000001209203,19.9999998790789)) ;
#5732=CARTESIAN_POINT('',(16.87,31.1,20.)) ;
#5733=CARTESIAN_POINT('',(10.0814213562,31.5100505063,20.)) ;
#5734=CARTESIAN_POINT('Origin',(11.0713699489153,32.4999986516766,19.9999984095466)) ;
#5735=CARTESIAN_POINT('',(8.49147186258,33.1,20.)) ;
#5736=CARTESIAN_POINT('',(9.28644660941,32.3050252532,20.)) ;
#5737=CARTESIAN_POINT('',(-8.49147186258,33.1,20.)) ;
#5738=CARTESIAN_POINT('',(3.5527136788E-14,33.1,20.)) ;
#5739=CARTESIAN_POINT('',(-10.0814213562,31.5100505063,20.)) ;
#5740=CARTESIAN_POINT('',(-9.28644660941,32.3050252532,20.)) ;
#5741=CARTESIAN_POINT('',(-11.0713708496686,31.100000074351,19.9999999256495)) ;
#5742=CARTESIAN_POINT('Origin',(-11.0713702946003,32.4999991690532,19.999999019805)) ;
#5743=CARTESIAN_POINT('',(-22.6686291501,31.1,20.)) ;
#5744=CARTESIAN_POINT('',(-16.87,31.1,20.)) ;
#5745=CARTESIAN_POINT('',(-23.6585785910206,31.5100505587523,19.9999999256531)) ;
#5746=CARTESIAN_POINT('Origin',(-22.6686293450353,32.4999990198376,19.9999990198396)) ;
#5747=CARTESIAN_POINT('',(-25.2485281374,33.1,20.)) ;
#5748=CARTESIAN_POINT('',(-24.4535533906,32.3050252532,20.)) ;
#5749=CARTESIAN_POINT('',(-42.7514718626,33.1,20.)) ;
#5750=CARTESIAN_POINT('',(-34.,33.1,20.)) ;
#5751=CARTESIAN_POINT('',(-44.4,31.4514718626,20.)) ;
#5752=CARTESIAN_POINT('',(-43.5757359313,32.2757359313,20.)) ;
#5753=CARTESIAN_POINT('',(-44.4,16.4985281374,20.)) ;
#5754=CARTESIAN_POINT('',(-44.4,23.975,20.)) ;
#5755=CARTESIAN_POINT('',(-42.2600505063,14.3585786438,20.)) ;
#5756=CARTESIAN_POINT('',(-43.3300252532,15.4285533906,20.)) ;
#5757=CARTESIAN_POINT('',(-41.8500000743509,13.3686291503314,19.9999999256495)) ;
#5758=CARTESIAN_POINT('Origin',(-43.2499991690533,13.3686297053997,19.9999990198052)) ;
#5759=CARTESIAN_POINT('',(-41.85,7.23431457505,20.)) ;
#5760=CARTESIAN_POINT('Origin',(43.2499999999937,13.3686291501029,19.6000000000109)) ;
#5761=CARTESIAN_POINT('',(42.45,13.3686291501,19.4)) ;
#5762=CARTESIAN_POINT('',(42.15,13.3686291501,19.7)) ;
#5763=CARTESIAN_POINT('',(42.6843145751,13.9343145751,19.4)) ;
#5764=CARTESIAN_POINT('Origin',(43.25,13.3686291501,19.4)) ;
#5765=CARTESIAN_POINT('',(42.4721825407,14.1464466094,19.7)) ;
#5766=CARTESIAN_POINT('Origin',(22.9057359313,-5.84426406871,19.4)) ;
#5767=CARTESIAN_POINT('',(44.8242640687,16.0742640687,19.4)) ;
#5768=CARTESIAN_POINT('',(43.165,14.415,19.4)) ;
#5769=CARTESIAN_POINT('',(44.6121320344,16.2863961031,19.7)) ;
#5770=CARTESIAN_POINT('Origin',(44.4,16.4985281374,18.9999999999991)) ;
#5771=CARTESIAN_POINT('',(45.,16.4985281374,19.4)) ;
#5772=CARTESIAN_POINT('Origin',(44.4,16.4985281374,19.4)) ;
#5773=CARTESIAN_POINT('',(44.7,16.4985281374,19.7)) ;
#5774=CARTESIAN_POINT('Origin',(45.,-5.42,19.4)) ;
#5775=CARTESIAN_POINT('',(45.,31.4514718626,19.4)) ;
#5776=CARTESIAN_POINT('',(45.,17.4,19.4)) ;
#5777=CARTESIAN_POINT('',(44.7,31.4514718626,19.7)) ;
#5778=CARTESIAN_POINT('Origin',(44.4,31.4514718626,18.9999999999991)) ;
#5779=CARTESIAN_POINT('',(44.8242640687,31.8757359313,19.4)) ;
#5780=CARTESIAN_POINT('Origin',(44.4,31.4514718626,19.4)) ;
#5781=CARTESIAN_POINT('',(44.6121320344,31.6636038969,19.7)) ;
#5782=CARTESIAN_POINT('Origin',(36.0557359313,40.6442640687,19.4)) ;
#5783=CARTESIAN_POINT('',(43.1757359313,33.5242640687,19.4)) ;
#5784=CARTESIAN_POINT('',(49.74,26.96,19.4)) ;
#5785=CARTESIAN_POINT('',(42.9636038969,33.3121320344,19.7)) ;
#5786=CARTESIAN_POINT('Origin',(42.7514718626,33.1,18.9999999999991)) ;
#5787=CARTESIAN_POINT('',(42.7514718626,33.7,19.4)) ;
#5788=CARTESIAN_POINT('Origin',(42.7514718626,33.1,19.4)) ;
#5789=CARTESIAN_POINT('',(42.7514718626,33.4,19.7)) ;
#5790=CARTESIAN_POINT('Origin',(-63.,33.7,19.4)) ;
#5791=CARTESIAN_POINT('',(25.2485281374,33.7,19.4)) ;
#5792=CARTESIAN_POINT('',(0.,33.7,19.4)) ;
#5793=CARTESIAN_POINT('',(25.2485281374,33.4,19.7)) ;
#5794=CARTESIAN_POINT('Origin',(25.2485281374,33.1,18.9999999999991)) ;
#5795=CARTESIAN_POINT('',(24.8242640687,33.5242640687,19.4)) ;
#5796=CARTESIAN_POINT('Origin',(25.2485281374,33.1,19.4)) ;
#5797=CARTESIAN_POINT('',(25.0363961031,33.3121320344,19.7)) ;
#5798=CARTESIAN_POINT('Origin',(-13.6957359313,-4.99573593129,19.4)) ;
#5799=CARTESIAN_POINT('',(23.2343145751,31.9343145751,19.4)) ;
#5800=CARTESIAN_POINT('',(9.12426406871,17.8242640687,19.4)) ;
#5801=CARTESIAN_POINT('',(23.4464466094,31.7221825407,19.7)) ;
#5802=CARTESIAN_POINT('Origin',(22.6686291501024,32.4999999999935,19.6000000000109)) ;
#5803=CARTESIAN_POINT('',(22.6686291501,31.7,19.4)) ;
#5804=CARTESIAN_POINT('Origin',(22.6686291501,32.5,19.4)) ;
#5805=CARTESIAN_POINT('',(22.6686291501,31.4,19.7)) ;
#5806=CARTESIAN_POINT('Origin',(-63.,31.7,19.4)) ;
#5807=CARTESIAN_POINT('',(11.0713708499,31.7,19.4)) ;
#5808=CARTESIAN_POINT('',(0.,31.7,19.4)) ;
#5809=CARTESIAN_POINT('',(11.0713708499,31.4,19.7)) ;
#5810=CARTESIAN_POINT('Origin',(11.0713708498971,32.4999999999937,19.6000000000109)) ;
#5811=CARTESIAN_POINT('',(10.5056854249,31.9343145751,19.4)) ;
#5812=CARTESIAN_POINT('Origin',(11.0713708499,32.5,19.4)) ;
#5813=CARTESIAN_POINT('',(10.2935533906,31.7221825407,19.7)) ;
#5814=CARTESIAN_POINT('Origin',(1.79573593129,40.6442640687,19.4)) ;
#5815=CARTESIAN_POINT('',(8.91573593129,33.5242640687,19.4)) ;
#5816=CARTESIAN_POINT('',(24.6157359313,17.8242640687,19.4)) ;
#5817=CARTESIAN_POINT('',(8.70360389693,33.3121320344,19.7)) ;
#5818=CARTESIAN_POINT('Origin',(8.49147186258,33.1,18.9999999999991)) ;
#5819=CARTESIAN_POINT('',(8.49147186258,33.7,19.4)) ;
#5820=CARTESIAN_POINT('Origin',(8.49147186258,33.1,19.4)) ;
#5821=CARTESIAN_POINT('',(8.49147186258,33.4,19.7)) ;
#5822=CARTESIAN_POINT('Origin',(-63.,33.7,19.4)) ;
#5823=CARTESIAN_POINT('',(-8.49147186258,33.7,19.4)) ;
#5824=CARTESIAN_POINT('',(0.,33.7,19.4)) ;
#5825=CARTESIAN_POINT('',(-8.49147186258,33.4,19.7)) ;
#5826=CARTESIAN_POINT('Origin',(-8.49147186258,33.1,18.9999999999991)) ;
#5827=CARTESIAN_POINT('',(-8.91573593129,33.5242640687,19.4)) ;
#5828=CARTESIAN_POINT('Origin',(-8.49147186258,33.1,19.4)) ;
#5829=CARTESIAN_POINT('',(-8.70360389693,33.3121320344,19.7)) ;
#5830=CARTESIAN_POINT('Origin',(-1.79573593129,40.6442640687,19.4)) ;
#5831=CARTESIAN_POINT('',(-10.5056854249,31.9343145751,19.4)) ;
#5832=CARTESIAN_POINT('',(-24.6157359313,17.8242640687,19.4)) ;
#5833=CARTESIAN_POINT('',(-10.2935533906,31.7221825407,19.7)) ;
#5834=CARTESIAN_POINT('Origin',(-11.0713708499,32.5,19.6000000000009)) ;
#5835=CARTESIAN_POINT('',(-11.0713708499,31.7,19.4)) ;
#5836=CARTESIAN_POINT('Origin',(-11.0713708499,32.5,19.4)) ;
#5837=CARTESIAN_POINT('',(-11.0713708499,31.4,19.7)) ;
#5838=CARTESIAN_POINT('Origin',(-63.,31.7,19.4)) ;
#5839=CARTESIAN_POINT('',(-22.6686291501,31.7,19.4)) ;
#5840=CARTESIAN_POINT('',(0.,31.7,19.4)) ;
#5841=CARTESIAN_POINT('',(-22.6686291501,31.4,19.7)) ;
#5842=CARTESIAN_POINT('Origin',(-22.6686291501,32.5,19.6000000000009)) ;
#5843=CARTESIAN_POINT('',(-23.2343145751,31.9343145751,19.4)) ;
#5844=CARTESIAN_POINT('Origin',(-22.6686291501,32.5,19.4)) ;
#5845=CARTESIAN_POINT('',(-23.4464466094,31.7221825407,19.7)) ;
#5846=CARTESIAN_POINT('Origin',(13.6957359313,-4.99573593129,19.4)) ;
#5847=CARTESIAN_POINT('',(-24.8242640687,33.5242640687,19.4)) ;
#5848=CARTESIAN_POINT('',(-9.12426406871,17.8242640687,19.4)) ;
#5849=CARTESIAN_POINT('',(-25.0363961031,33.3121320344,19.7)) ;
#5850=CARTESIAN_POINT('Origin',(-25.2485281374,33.1000000000001,18.9999999999991)) ;
#5851=CARTESIAN_POINT('',(-25.2485281374,33.7,19.4)) ;
#5852=CARTESIAN_POINT('Origin',(-25.2485281374,33.1,19.4)) ;
#5853=CARTESIAN_POINT('',(-25.2485281374,33.4,19.7)) ;
#5854=CARTESIAN_POINT('Origin',(-63.,33.7,19.4)) ;
#5855=CARTESIAN_POINT('',(-42.7514718626,33.7,19.4)) ;
#5856=CARTESIAN_POINT('',(0.,33.7,19.4)) ;
#5857=CARTESIAN_POINT('',(-42.7514718626,33.4,19.7)) ;
#5858=CARTESIAN_POINT('Origin',(-42.7514718626,33.1,18.9999999999991)) ;
#5859=CARTESIAN_POINT('',(-43.1757359313,33.5242640687,19.4)) ;
#5860=CARTESIAN_POINT('Origin',(-42.7514718626,33.1,19.4)) ;
#5861=CARTESIAN_POINT('',(-42.9636038969,33.3121320344,19.7)) ;
#5862=CARTESIAN_POINT('Origin',(-43.1757359313,33.5242640687,19.4)) ;
#5863=CARTESIAN_POINT('',(-44.8242640687,31.8757359313,19.4)) ;
#5864=CARTESIAN_POINT('',(-53.3,23.4,19.4)) ;
#5865=CARTESIAN_POINT('',(-44.6121320344,31.6636038969,19.7)) ;
#5866=CARTESIAN_POINT('Origin',(-44.4,31.4514718626,18.9999999999991)) ;
#5867=CARTESIAN_POINT('',(-45.,31.4514718626,19.4)) ;
#5868=CARTESIAN_POINT('Origin',(-44.4,31.4514718626,19.4)) ;
#5869=CARTESIAN_POINT('',(-44.7,31.4514718626,19.7)) ;
#5870=CARTESIAN_POINT('Origin',(-45.,-5.42,19.4)) ;
#5871=CARTESIAN_POINT('',(-45.,16.4985281374,19.4)) ;
#5872=CARTESIAN_POINT('',(-45.,17.4,19.4)) ;
#5873=CARTESIAN_POINT('',(-44.7,16.4985281374,19.7)) ;
#5874=CARTESIAN_POINT('Origin',(-44.4,16.4985281374,18.9999999999991)) ;
#5875=CARTESIAN_POINT('',(-44.8242640687,16.0742640687,19.4)) ;
#5876=CARTESIAN_POINT('Origin',(-44.4,16.4985281374,19.4)) ;
#5877=CARTESIAN_POINT('',(-44.6121320344,16.2863961031,19.7)) ;
#5878=CARTESIAN_POINT('Origin',(-22.9057359313,-5.84426406871,19.4)) ;
#5879=CARTESIAN_POINT('',(-42.6843145751,13.9343145751,19.4)) ;
#5880=CARTESIAN_POINT('',(-33.865,5.115,19.4)) ;
#5881=CARTESIAN_POINT('',(-42.4721825407,14.1464466094,19.7)) ;
#5882=CARTESIAN_POINT('Origin',(-43.25,13.3686291501,19.6000000000009)) ;
#5883=CARTESIAN_POINT('',(-42.45,13.3686291501,19.4)) ;
#5884=CARTESIAN_POINT('Origin',(-43.25,13.3686291501,19.4)) ;
#5885=CARTESIAN_POINT('',(-42.15,13.3686291501,19.7)) ;
#5886=CARTESIAN_POINT('Origin',(-42.45,-5.42,19.4)) ;
#5887=CARTESIAN_POINT('',(-42.45,1.1,19.4)) ;
#5888=CARTESIAN_POINT('',(-42.15,1.1,19.7)) ;
#5889=CARTESIAN_POINT('',(-42.45,3.97431457505,19.4)) ;
#5890=CARTESIAN_POINT('Origin',(42.45,-5.42,19.4)) ;
#5891=CARTESIAN_POINT('',(42.45,1.1,19.4)) ;
#5892=CARTESIAN_POINT('',(42.45,17.4,19.4)) ;
#5893=CARTESIAN_POINT('',(42.15,1.1,19.7)) ;
#5894=CARTESIAN_POINT('Origin',(0.,0.,-20.)) ;
#5895=CARTESIAN_POINT('',(-41.8500000743509,13.3686292513994,-19.9999999256495)) ;
#5896=CARTESIAN_POINT('',(-41.85,1.1,-20.)) ;
#5897=CARTESIAN_POINT('',(-41.85,7.23431457505,-20.)) ;
#5898=CARTESIAN_POINT('',(-42.2600505063,14.3585786438,-20.)) ;
#5899=CARTESIAN_POINT('Origin',(-43.2499991690534,13.3686297053996,-19.9999990198051)) ;
#5900=CARTESIAN_POINT('',(-44.4,16.4985281374,-20.)) ;
#5901=CARTESIAN_POINT('',(-43.3300252532,15.4285533906,-20.)) ;
#5902=CARTESIAN_POINT('',(-44.4,31.4514718626,-20.)) ;
#5903=CARTESIAN_POINT('',(-44.4,23.975,-20.)) ;
#5904=CARTESIAN_POINT('',(-42.7514718626,33.1,-20.)) ;
#5905=CARTESIAN_POINT('',(-43.5757359313,32.2757359313,-20.)) ;
#5906=CARTESIAN_POINT('',(-25.2485281374,33.1,-20.)) ;
#5907=CARTESIAN_POINT('',(-34.,33.1,-20.)) ;
#5908=CARTESIAN_POINT('',(-23.6585785195402,31.510050487272,-19.9999999256531)) ;
#5909=CARTESIAN_POINT('',(-24.4535533906,32.3050252532,-20.)) ;
#5910=CARTESIAN_POINT('',(-22.6686291501,31.1,-20.)) ;
#5911=CARTESIAN_POINT('Origin',(-22.6686293450353,32.4999990198376,-19.9999990198394)) ;
#5912=CARTESIAN_POINT('',(-11.0713707486006,31.1000000743509,-19.9999999256495)) ;
#5913=CARTESIAN_POINT('',(-16.87,31.1,-20.)) ;
#5914=CARTESIAN_POINT('',(-10.0814213562,31.5100505063,-20.)) ;
#5915=CARTESIAN_POINT('Origin',(-11.0713702946003,32.4999991690532,-19.999999019805)) ;
#5916=CARTESIAN_POINT('',(-8.49147186258,33.1,-20.)) ;
#5917=CARTESIAN_POINT('',(-9.28644660941,32.3050252532,-20.)) ;
#5918=CARTESIAN_POINT('',(8.49147186258,33.1,-20.)) ;
#5919=CARTESIAN_POINT('',(2.48689957516E-14,33.1,-20.)) ;
#5920=CARTESIAN_POINT('',(10.0814213562,31.5100505063,-20.)) ;
#5921=CARTESIAN_POINT('',(9.28644660941,32.3050252532,-20.)) ;
#5922=CARTESIAN_POINT('',(11.0713708500427,31.1000001209198,-19.9999998790785)) ;
#5923=CARTESIAN_POINT('Origin',(11.071369948907,32.4999986516472,-19.9999984095746)) ;
#5924=CARTESIAN_POINT('',(22.6686291501,31.1,-20.)) ;
#5925=CARTESIAN_POINT('',(16.87,31.1,-20.)) ;
#5926=CARTESIAN_POINT('',(23.6585785583635,31.5100505919384,-19.9999998790928)) ;
#5927=CARTESIAN_POINT('Origin',(22.6686294664411,32.4999984096401,-19.9999984097149)) ;
#5928=CARTESIAN_POINT('',(25.2485281374,33.1,-20.)) ;
#5929=CARTESIAN_POINT('',(24.4535533906,32.3050252532,-20.)) ;
#5930=CARTESIAN_POINT('',(42.7514718626,33.1,-20.)) ;
#5931=CARTESIAN_POINT('',(34.,33.1,-20.)) ;
#5932=CARTESIAN_POINT('',(44.4,31.4514718626,-20.)) ;
#5933=CARTESIAN_POINT('',(43.5757359313,32.2757359313,-20.)) ;
#5934=CARTESIAN_POINT('',(44.4,16.4985281374,-20.)) ;
#5935=CARTESIAN_POINT('',(44.4,23.975,-20.)) ;
#5936=CARTESIAN_POINT('',(42.2600505063,14.3585786438,-20.)) ;
#5937=CARTESIAN_POINT('',(43.3300252532,15.4285533906,-20.)) ;
#5938=CARTESIAN_POINT('',(41.8500001209206,13.3686289388372,-19.9999998790791)) ;
#5939=CARTESIAN_POINT('Origin',(43.2499986516453,13.3686300510977,-19.9999984095153)) ;
#5940=CARTESIAN_POINT('',(41.85,1.1,-20.)) ;
#5941=CARTESIAN_POINT('',(41.85,7.23431457505,-20.)) ;
#5942=CARTESIAN_POINT('',(35.1643820091,1.1,-20.)) ;
#5943=CARTESIAN_POINT('',(-35.1643820091,1.1,-20.)) ;
#5944=CARTESIAN_POINT('Origin',(22.6686291501,32.5,0.)) ;
#5945=CARTESIAN_POINT('',(23.2343145751,31.9343145751,-19.4)) ;
#5946=CARTESIAN_POINT('',(22.6686291501,31.7,-19.4)) ;
#5947=CARTESIAN_POINT('Origin',(22.6686291501,32.5,-19.4)) ;
#5948=CARTESIAN_POINT('',(22.6686291501,31.7,0.)) ;
#5949=CARTESIAN_POINT('',(23.2343145751,31.9343145751,0.)) ;
#5950=CARTESIAN_POINT('Origin',(11.0713708499,32.5,0.)) ;
#5951=CARTESIAN_POINT('',(11.0713708499,31.7,-19.4)) ;
#5952=CARTESIAN_POINT('',(10.5056854249,31.9343145751,-19.4)) ;
#5953=CARTESIAN_POINT('Origin',(11.0713708499,32.5,-19.4)) ;
#5954=CARTESIAN_POINT('',(10.5056854249,31.9343145751,0.)) ;
#5955=CARTESIAN_POINT('',(11.0713708499,31.7,0.)) ;
#5956=CARTESIAN_POINT('Origin',(-11.0713708499,32.5,0.)) ;
#5957=CARTESIAN_POINT('',(-10.5056854249,31.9343145751,-19.4)) ;
#5958=CARTESIAN_POINT('',(-11.0713708211758,31.7,-19.4)) ;
#5959=CARTESIAN_POINT('Origin',(-11.0713708499,32.5,-19.4)) ;
#5960=CARTESIAN_POINT('',(-11.0713708499,31.7,0.)) ;
#5961=CARTESIAN_POINT('',(-10.5056854249,31.9343145751,0.)) ;
#5962=CARTESIAN_POINT('Origin',(-22.6686291501,32.5,0.)) ;
#5963=CARTESIAN_POINT('',(-22.6686291501,31.7,-19.4)) ;
#5964=CARTESIAN_POINT('',(-23.2343145547562,31.934314554758,-19.4000000000014)) ;
#5965=CARTESIAN_POINT('Origin',(-22.6686291501,32.5,-19.4)) ;
#5966=CARTESIAN_POINT('',(-23.2343145751,31.9343145751,0.)) ;
#5967=CARTESIAN_POINT('',(-22.6686291501,31.7,0.)) ;
#5968=CARTESIAN_POINT('Origin',(-43.25,13.3686291501,0.)) ;
#5969=CARTESIAN_POINT('',(-42.6843145751,13.9343145751,-19.4)) ;
#5970=CARTESIAN_POINT('',(-42.45,13.3686291788242,-19.4)) ;
#5971=CARTESIAN_POINT('Origin',(-43.25,13.3686291501,-19.4)) ;
#5972=CARTESIAN_POINT('',(-42.45,13.3686291501,0.)) ;
#5973=CARTESIAN_POINT('',(-42.6843145751,13.9343145751,0.)) ;
#5974=CARTESIAN_POINT('Origin',(43.25,13.3686291501,0.)) ;
#5975=CARTESIAN_POINT('',(42.4499999999998,13.3686290899674,-19.3999999999998)) ;
#5976=CARTESIAN_POINT('',(42.6843145751,13.9343145751,-19.4)) ;
#5977=CARTESIAN_POINT('Origin',(43.25,13.3686291501,-19.4)) ;
#5978=CARTESIAN_POINT('',(42.6843145751,13.9343145751,0.)) ;
#5979=CARTESIAN_POINT('',(42.45,13.3686291501,0.)) ;
#5980=CARTESIAN_POINT('Origin',(42.45,13.7,0.)) ;
#5981=CARTESIAN_POINT('',(42.45,1.1,-19.4)) ;
#5982=CARTESIAN_POINT('',(42.45,7.23431457505,-19.4)) ;
#5983=CARTESIAN_POINT('',(42.45,1.1,0.)) ;
#5984=CARTESIAN_POINT('Origin',(23.,31.7,0.)) ;
#5985=CARTESIAN_POINT('',(-16.87,31.7,-19.4)) ;
#5986=CARTESIAN_POINT('Origin',(23.,31.7,0.)) ;
#5987=CARTESIAN_POINT('',(16.87,31.7,-19.4)) ;
#5988=CARTESIAN_POINT('Origin',(-42.45,13.7,0.)) ;
#5989=CARTESIAN_POINT('',(-42.45,1.1,-19.4)) ;
#5990=CARTESIAN_POINT('',(-42.45,1.1,0.)) ;
#5991=CARTESIAN_POINT('',(-42.45,7.23431457505,-19.4)) ;
#5992=CARTESIAN_POINT('Origin',(-42.45,1.1,0.)) ;
#5993=CARTESIAN_POINT('',(42.15,1.1,-19.7)) ;
#5994=CARTESIAN_POINT('Origin',(-42.45,1.1,0.)) ;
#5995=CARTESIAN_POINT('',(-42.15,1.1,-19.7)) ;
#5996=CARTESIAN_POINT('Origin',(44.4,31.4514718626,0.)) ;
#5997=CARTESIAN_POINT('',(44.8242640687,31.8757359313,-19.4)) ;
#5998=CARTESIAN_POINT('',(44.8242640687,31.8757359313,0.)) ;
#5999=CARTESIAN_POINT('',(45.,31.4514718626,-19.4)) ;
#6000=CARTESIAN_POINT('',(45.,31.4514718626,0.)) ;
#6001=CARTESIAN_POINT('Origin',(44.4,31.4514718626,-19.4)) ;
#6002=CARTESIAN_POINT('Origin',(45.,31.7,0.)) ;
#6003=CARTESIAN_POINT('',(43.1757359313,33.5242640687,-19.4)) ;
#6004=CARTESIAN_POINT('',(43.1757359313,33.5242640687,0.)) ;
#6005=CARTESIAN_POINT('',(44.,32.7,-19.4)) ;
#6006=CARTESIAN_POINT('Origin',(42.7514718626,33.1,0.)) ;
#6007=CARTESIAN_POINT('',(42.7514718626,33.7,-19.4)) ;
#6008=CARTESIAN_POINT('',(42.7514718626,33.7,0.)) ;
#6009=CARTESIAN_POINT('Origin',(42.7514718626,33.1,-19.4)) ;
#6010=CARTESIAN_POINT('Origin',(25.,33.7,0.)) ;
#6011=CARTESIAN_POINT('',(24.8242640687,33.5242640687,-19.4)) ;
#6012=CARTESIAN_POINT('',(24.8242640687,33.5242640687,0.)) ;
#6013=CARTESIAN_POINT('',(24.0292893219,32.7292893219,-19.4)) ;
#6014=CARTESIAN_POINT('Origin',(43.,33.7,0.)) ;
#6015=CARTESIAN_POINT('',(25.2485281374,33.7,-19.4)) ;
#6016=CARTESIAN_POINT('',(25.2485281374,33.7,0.)) ;
#6017=CARTESIAN_POINT('',(34.,33.7,-19.4)) ;
#6018=CARTESIAN_POINT('Origin',(25.2485281374,33.1,0.)) ;
#6019=CARTESIAN_POINT('Origin',(25.2485281374,33.1,-19.4)) ;
#6020=CARTESIAN_POINT('Origin',(10.74,31.7,0.)) ;
#6021=CARTESIAN_POINT('',(8.91573593129,33.5242640687,-19.4)) ;
#6022=CARTESIAN_POINT('',(8.91573593129,33.5242640687,0.)) ;
#6023=CARTESIAN_POINT('',(9.71071067812,32.7292893219,-19.4)) ;
#6024=CARTESIAN_POINT('Origin',(8.49147186258,33.1,0.)) ;
#6025=CARTESIAN_POINT('',(8.49147186258,33.7,-19.4)) ;
#6026=CARTESIAN_POINT('',(8.49147186258,33.7,0.)) ;
#6027=CARTESIAN_POINT('Origin',(8.49147186258,33.1,-19.4)) ;
#6028=CARTESIAN_POINT('Origin',(-10.74,31.7,0.)) ;
#6029=CARTESIAN_POINT('',(-8.91573593129,33.5242640687,-19.4)) ;
#6030=CARTESIAN_POINT('',(-9.71071067812,32.7292893219,-19.4)) ;
#6031=CARTESIAN_POINT('',(-8.91573593129,33.5242640687,0.)) ;
#6032=CARTESIAN_POINT('Origin',(43.,33.7,0.)) ;
#6033=CARTESIAN_POINT('',(-8.49147186258,33.7,-19.4)) ;
#6034=CARTESIAN_POINT('',(-8.49147186258,33.7,0.)) ;
#6035=CARTESIAN_POINT('',(0.,33.7,-19.4)) ;
#6036=CARTESIAN_POINT('Origin',(-8.49147186258,33.1,0.)) ;
#6037=CARTESIAN_POINT('Origin',(-8.49147186258,33.1,-19.4)) ;
#6038=CARTESIAN_POINT('Origin',(-25.,33.7,0.)) ;
#6039=CARTESIAN_POINT('',(-24.8242640687,33.5242640687,-19.4)) ;
#6040=CARTESIAN_POINT('',(-24.0292893219,32.7292893219,-19.4)) ;
#6041=CARTESIAN_POINT('',(-24.8242640687,33.5242640687,0.)) ;
#6042=CARTESIAN_POINT('Origin',(-25.2485281374,33.1,0.)) ;
#6043=CARTESIAN_POINT('',(-25.2485281374,33.7,-19.4)) ;
#6044=CARTESIAN_POINT('',(-25.2485281374,33.7,0.)) ;
#6045=CARTESIAN_POINT('Origin',(-25.2485281374,33.1,-19.4)) ;
#6046=CARTESIAN_POINT('Origin',(43.,33.7,0.)) ;
#6047=CARTESIAN_POINT('',(-42.7514718626,33.7,-19.4)) ;
#6048=CARTESIAN_POINT('',(-42.7514718626,33.7,0.)) ;
#6049=CARTESIAN_POINT('',(-34.,33.7,-19.4)) ;
#6050=CARTESIAN_POINT('Origin',(-42.7514718626,33.1,0.)) ;
#6051=CARTESIAN_POINT('',(-43.1757359313,33.5242640687,-19.4)) ;
#6052=CARTESIAN_POINT('',(-43.1757359313,33.5242640687,0.)) ;
#6053=CARTESIAN_POINT('Origin',(-42.7514718626,33.1,-19.4)) ;
#6054=CARTESIAN_POINT('Origin',(-45.,31.7,0.)) ;
#6055=CARTESIAN_POINT('',(-44.8242640687,31.8757359313,-19.4)) ;
#6056=CARTESIAN_POINT('',(-44.,32.7,-19.4)) ;
#6057=CARTESIAN_POINT('',(-44.8242640687,31.8757359313,0.)) ;
#6058=CARTESIAN_POINT('Origin',(-44.4,31.4514718626,0.)) ;
#6059=CARTESIAN_POINT('',(-45.,31.4514718626,-19.4)) ;
#6060=CARTESIAN_POINT('',(-45.,31.4514718626,0.)) ;
#6061=CARTESIAN_POINT('Origin',(-44.4,31.4514718626,-19.4)) ;
#6062=CARTESIAN_POINT('Origin',(45.,16.25,0.)) ;
#6063=CARTESIAN_POINT('',(44.8242640687,16.0742640687,-19.4)) ;
#6064=CARTESIAN_POINT('',(43.7542893219,15.0042893219,-19.4)) ;
#6065=CARTESIAN_POINT('',(44.8242640687,16.0742640687,0.)) ;
#6066=CARTESIAN_POINT('Origin',(45.,31.7,0.)) ;
#6067=CARTESIAN_POINT('',(45.,16.4985281374,-19.4)) ;
#6068=CARTESIAN_POINT('',(45.,23.975,-19.4)) ;
#6069=CARTESIAN_POINT('',(45.,16.4985281374,0.)) ;
#6070=CARTESIAN_POINT('Origin',(44.4,16.4985281374,0.)) ;
#6071=CARTESIAN_POINT('Origin',(44.4,16.4985281374,-19.4)) ;
#6072=CARTESIAN_POINT('Origin',(-45.,16.25,0.)) ;
#6073=CARTESIAN_POINT('',(-44.8242640687,16.0742640687,-19.4)) ;
#6074=CARTESIAN_POINT('',(-44.8242640687,16.0742640687,0.)) ;
#6075=CARTESIAN_POINT('',(-43.7542893219,15.0042893219,-19.4)) ;
#6076=CARTESIAN_POINT('Origin',(-45.,31.7,0.)) ;
#6077=CARTESIAN_POINT('',(-45.,16.4985281374,-19.4)) ;
#6078=CARTESIAN_POINT('',(-45.,16.4985281374,0.)) ;
#6079=CARTESIAN_POINT('',(-45.,23.975,-19.4)) ;
#6080=CARTESIAN_POINT('Origin',(-44.4,16.4985281374,0.)) ;
#6081=CARTESIAN_POINT('Origin',(-44.4,16.4985281374,-19.4)) ;
#6082=CARTESIAN_POINT('Origin',(43.2499999999937,13.3686291501029,-19.6000000000109)) ;
#6083=CARTESIAN_POINT('',(42.15,13.3686289841,-19.7)) ;
#6084=CARTESIAN_POINT('',(42.4721825407,14.1464466094,-19.7)) ;
#6085=CARTESIAN_POINT('Origin',(22.9057359313,-5.84426406871,-19.4)) ;
#6086=CARTESIAN_POINT('',(44.6121320344,16.2863961031,-19.7)) ;
#6087=CARTESIAN_POINT('Origin',(44.4,16.4985281374,-18.9999999999991)) ;
#6088=CARTESIAN_POINT('',(44.7,16.4985281374,-19.7)) ;
#6089=CARTESIAN_POINT('Origin',(45.,-5.42,-19.4)) ;
#6090=CARTESIAN_POINT('',(44.7,31.4514718626,-19.7)) ;
#6091=CARTESIAN_POINT('Origin',(44.4,31.4514718626,-18.9999999999991)) ;
#6092=CARTESIAN_POINT('',(44.6121320344,31.6636038969,-19.7)) ;
#6093=CARTESIAN_POINT('Origin',(36.0557359313,40.6442640687,-19.4)) ;
#6094=CARTESIAN_POINT('',(42.9636038969,33.3121320344,-19.7)) ;
#6095=CARTESIAN_POINT('Origin',(42.7514718626,33.1,-18.9999999999991)) ;
#6096=CARTESIAN_POINT('',(42.7514718626,33.4,-19.7)) ;
#6097=CARTESIAN_POINT('Origin',(-63.,33.7,-19.4)) ;
#6098=CARTESIAN_POINT('',(25.2485281374,33.4,-19.7)) ;
#6099=CARTESIAN_POINT('Origin',(25.2485281374,33.1,-18.9999999999991)) ;
#6100=CARTESIAN_POINT('',(25.0363961031,33.3121320344,-19.7)) ;
#6101=CARTESIAN_POINT('Origin',(-13.6957359313,-4.99573593129,-19.4)) ;
#6102=CARTESIAN_POINT('',(23.4464466094,31.7221825407,-19.7)) ;
#6103=CARTESIAN_POINT('Origin',(22.668629150113,32.4999999999744,-19.6000000000509)) ;
#6104=CARTESIAN_POINT('',(22.6686291501,31.4,-19.7)) ;
#6105=CARTESIAN_POINT('Origin',(-63.,31.7,-19.4)) ;
#6106=CARTESIAN_POINT('',(11.0713708499,31.4,-19.7)) ;
#6107=CARTESIAN_POINT('Origin',(11.0713708498911,32.4999999999727,-19.6000000000509)) ;
#6108=CARTESIAN_POINT('',(10.2935533906,31.7221825407,-19.7)) ;
#6109=CARTESIAN_POINT('Origin',(8.91573593129,33.5242640687,-19.4)) ;
#6110=CARTESIAN_POINT('',(8.70360389693,33.3121320344,-19.7)) ;
#6111=CARTESIAN_POINT('Origin',(8.49147186258,33.1,-18.9999999999991)) ;
#6112=CARTESIAN_POINT('',(8.49147186258,33.4,-19.7)) ;
#6113=CARTESIAN_POINT('Origin',(-63.,33.7,-19.4)) ;
#6114=CARTESIAN_POINT('',(-8.49147186258,33.4,-19.7)) ;
#6115=CARTESIAN_POINT('Origin',(-8.49147186258,33.1,-18.9999999999991)) ;
#6116=CARTESIAN_POINT('',(-8.70360389693,33.3121320344,-19.7)) ;
#6117=CARTESIAN_POINT('Origin',(-1.79573593129,40.6442640687,-19.4)) ;
#6118=CARTESIAN_POINT('',(-10.2935533906,31.7221825407,-19.7)) ;
#6119=CARTESIAN_POINT('Origin',(-11.0713708499,32.5,-19.6000000000009)) ;
#6120=CARTESIAN_POINT('',(-11.0713707703,31.4,-19.7)) ;
#6121=CARTESIAN_POINT('Origin',(-63.,31.7,-19.4)) ;
#6122=CARTESIAN_POINT('',(-22.6686291501,31.4,-19.7)) ;
#6123=CARTESIAN_POINT('Origin',(-22.6686291501,32.5,-19.6000000000009)) ;
#6124=CARTESIAN_POINT('',(-23.4464465531,31.7221824844,-19.7)) ;
#6125=CARTESIAN_POINT('Origin',(13.6957359313,-4.99573593129,-19.4)) ;
#6126=CARTESIAN_POINT('',(-25.0363961031,33.3121320344,-19.7)) ;
#6127=CARTESIAN_POINT('Origin',(-25.2485281374,33.1,-18.9999999999991)) ;
#6128=CARTESIAN_POINT('',(-25.2485281374,33.4,-19.7)) ;
#6129=CARTESIAN_POINT('Origin',(-63.,33.7,-19.4)) ;
#6130=CARTESIAN_POINT('',(-42.7514718626,33.4,-19.7)) ;
#6131=CARTESIAN_POINT('Origin',(-42.7514718626,33.1,-18.9999999999991)) ;
#6132=CARTESIAN_POINT('',(-42.9636038969,33.3121320344,-19.7)) ;
#6133=CARTESIAN_POINT('Origin',(-36.0557359313,40.6442640687,-19.4)) ;
#6134=CARTESIAN_POINT('',(-44.6121320344,31.6636038969,-19.7)) ;
#6135=CARTESIAN_POINT('Origin',(-44.4,31.4514718626,-18.9999999999991)) ;
#6136=CARTESIAN_POINT('',(-44.7,31.4514718626,-19.7)) ;
#6137=CARTESIAN_POINT('Origin',(-45.,-5.42,-19.4)) ;
#6138=CARTESIAN_POINT('',(-44.7,16.4985281374,-19.7)) ;
#6139=CARTESIAN_POINT('Origin',(-44.4,16.4985281374,-18.9999999999991)) ;
#6140=CARTESIAN_POINT('',(-44.6121320344,16.2863961031,-19.7)) ;
#6141=CARTESIAN_POINT('Origin',(-22.9057359313,-5.84426406871,-19.4)) ;
#6142=CARTESIAN_POINT('',(-42.4721825407,14.1464466094,-19.7)) ;
#6143=CARTESIAN_POINT('Origin',(-43.25,13.3686291501,-19.6000000000009)) ;
#6144=CARTESIAN_POINT('',(-42.15,13.3686292297,-19.7)) ;
#6145=CARTESIAN_POINT('Origin',(-42.45,-5.42,-19.4)) ;
#6146=CARTESIAN_POINT('Origin',(42.45,-5.42,-19.4)) ;
#6757=UNCERTAINTY_MEASURE_WITH_UNIT(LENGTH_MEASURE(0.01),#6780,
'DISTANCE_ACCURACY_VALUE',
'Maximum model space distance between geometric entities at asserted c
onnectivities') ;
#6767=UNCERTAINTY_MEASURE_WITH_UNIT(LENGTH_MEASURE(0.01),#6780,
'DISTANCE_ACCURACY_VALUE',
'Maximum model space distance between geometric entities at asserted c
onnectivities') ;
#6769=(
GEOMETRIC_REPRESENTATION_CONTEXT(3)
GLOBAL_UNCERTAINTY_ASSIGNED_CONTEXT((#6757))
GLOBAL_UNIT_ASSIGNED_CONTEXT((#6780,#6782,#6783))
REPRESENTATION_CONTEXT('','3D')
) ;
#6779=(
GEOMETRIC_REPRESENTATION_CONTEXT(3)
GLOBAL_UNCERTAINTY_ASSIGNED_CONTEXT((#6767))
GLOBAL_UNIT_ASSIGNED_CONTEXT((#6780,#6782,#6783))
REPRESENTATION_CONTEXT('','3D')
) ;
#6780=(
LENGTH_UNIT()
NAMED_UNIT(*)
SI_UNIT(.MILLI.,.METRE.)
) ;
#6782=(
NAMED_UNIT(*)
PLANE_ANGLE_UNIT()
SI_UNIT($,.RADIAN.)
) ;
#6783=(
NAMED_UNIT(*)
SI_UNIT($,.STERADIAN.)
SOLID_ANGLE_UNIT()
) ;
#6785=SHAPE_DEFINITION_REPRESENTATION(#6796,#6817) ;
#6796=PRODUCT_DEFINITION_SHAPE('',$,#6829) ;
#6817=SHAPE_REPRESENTATION('',(#4017),#6769) ;
#6827=PRODUCT_DEFINITION_CONTEXT('part definition',#6862,'design') ;
#6829=PRODUCT_DEFINITION('Clamp_Body_Upper','Clamp_Body_Upper',#6840,#6827) ;
#6840=PRODUCT_DEFINITION_FORMATION('',$,#6865) ;
#6862=APPLICATION_CONTEXT(
'Core Data for Automotive Mechanical Design Process') ;
#6863=PRODUCT_CONTEXT('part definition',#6862,'mechanical') ;
#6865=PRODUCT('Clamp_Body_Upper','Clamp_Body_Upper',$,(#6863)) ;
#6876=PRESENTATION_STYLE_ASSIGNMENT((#6879)) ;
#6879=SURFACE_STYLE_USAGE(.BOTH.,#6882) ;
#6882=SURFACE_SIDE_STYLE('',(#6885)) ;
#6885=SURFACE_STYLE_FILL_AREA(#6888) ;
#6888=FILL_AREA_STYLE('Opaque(245,245,246)',(#6891)) ;
#6891=FILL_AREA_STYLE_COLOUR('Opaque(245,245,246)',#6894) ;
#6894=COLOUR_RGB('Opaque(245,245,246)', 0.09019608, 0.27058824, 0.51372549) ;
ENDSEC;
END-ISO-10303-21;
